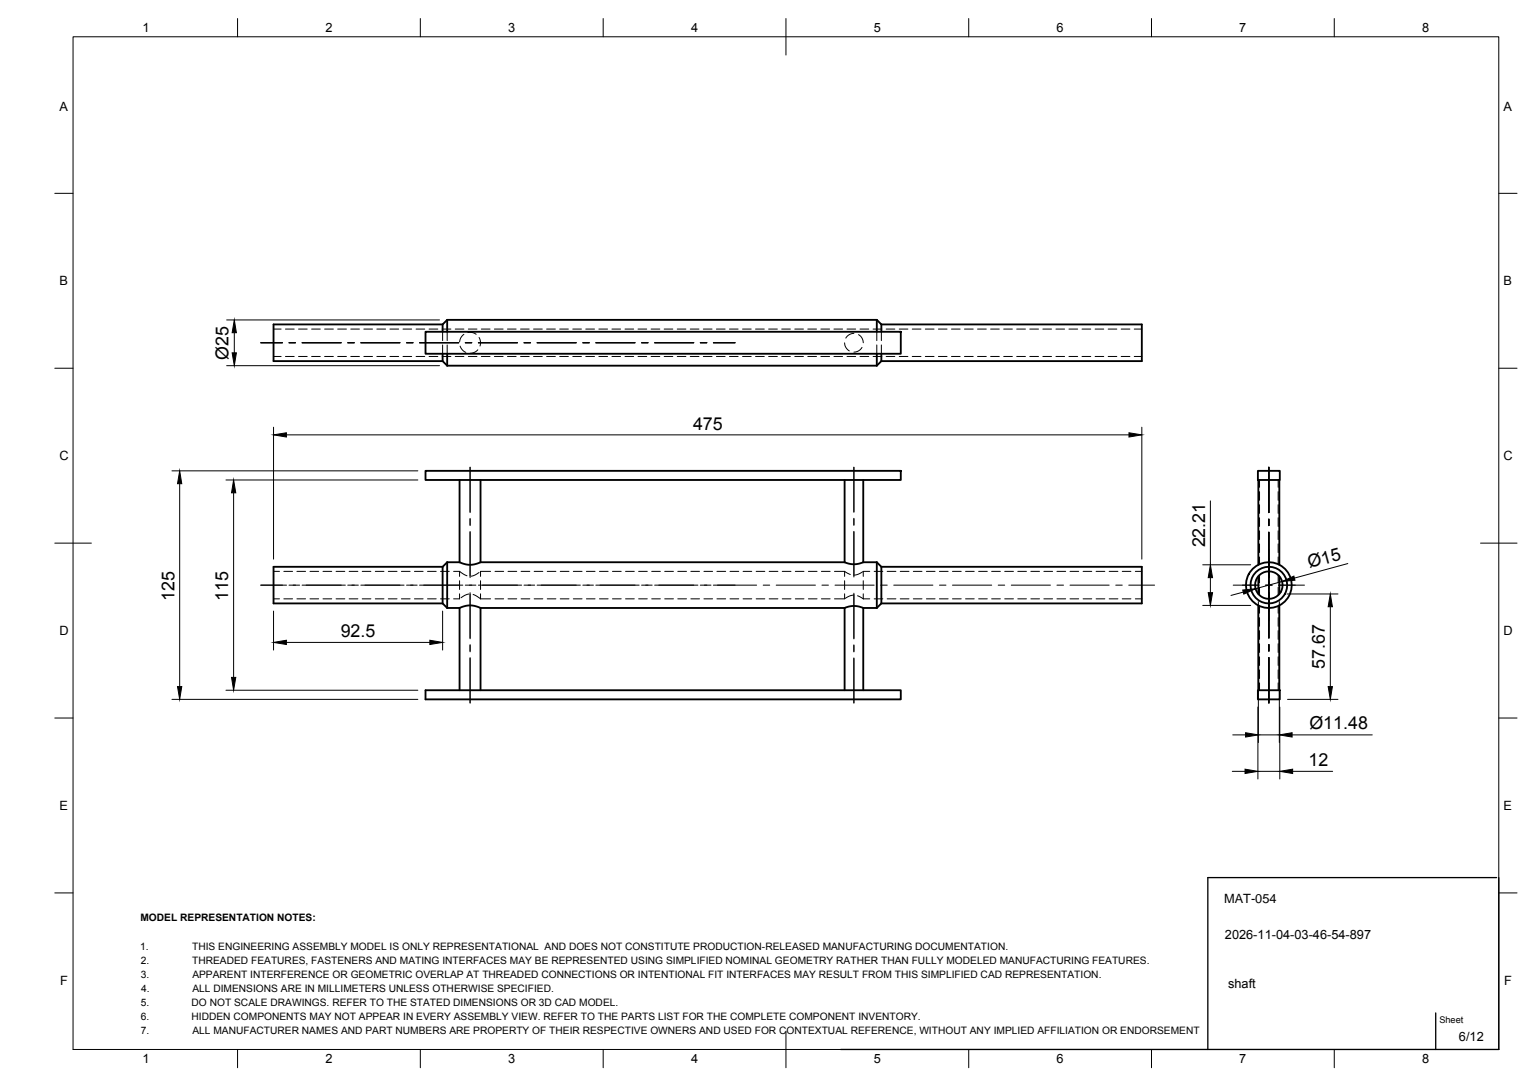
ISO-10303-21;
HEADER;
FILE_DESCRIPTION (('STEP AP214'),
    '1' );
FILE_NAME ('shaft.step',
    '2026-10-21T17:50:41',
    ( '' ),
    ( '' ),
    'SwSTEP 2.0',
    'SolidWorks 2026',
    '' );
FILE_SCHEMA (( 'AUTOMOTIVE_DESIGN' ));
ENDSEC;

DATA;
#16=VERTEX_POINT ( 'NONE', #3282 ) ;
#58=ADVANCED_FACE ( 'NONE', ( #14158 ), #33712, .T. ) ;
#109=VERTEX_POINT ( 'NONE', #18069 ) ;
#119=LINE ( 'NONE', #24139, #24170 ) ;
#137=CARTESIAN_POINT ( 'NONE',  ( -110.0810685637187021, 0.6776097359754142957, -12.48599830169775871 ) ) ;
#156=CARTESIAN_POINT ( 'NONE',  ( -109.6397584259853915, -2.159755022470678298, 7.184107906894084294 ) ) ;
#175=EDGE_CURVE ( 'NONE', #17916, #26514, #22520, .T. ) ;
#187=CIRCLE ( 'NONE', #747, 5.738084889453667792 ) ;
#195=ORIENTED_EDGE ( 'NONE', *, *, #25088, .F. ) ;
#198=CARTESIAN_POINT ( 'NONE',  ( 105.9801405217367147, 5.657025933901884684, 4.924586583110066584 ) ) ;
#251=ORIENTED_EDGE ( 'NONE', *, *, #8791, .F. ) ;
#257=CARTESIAN_POINT ( 'NONE',  ( 106.5104497542385928, -5.548707632555109015, -11.20129239819138967 ) ) ;
#273=EDGE_CURVE ( 'NONE', #17170, #26514, #10910, .T. ) ;
#275=CARTESIAN_POINT ( 'NONE',  ( -130.6469666100234406, 6.000000000000000000, 57.49999999999999289 ) ) ;
#291=CARTESIAN_POINT ( 'NONE',  ( -101.1657792522907329, 3.400963087932908024, 6.689628992625340942 ) ) ;
#341=CARTESIAN_POINT ( 'NONE',  ( -103.3057560645484045, -4.837552664684794834, 5.733718144795171945 ) ) ;
#348=VECTOR ( 'NONE', #16267, 1000.000000000000000 ) ;
#350=CARTESIAN_POINT ( 'NONE',  ( 105.0000000000000000, 0.000000000000000000, 60.00000000000000000 ) ) ;
#375=ORIENTED_EDGE ( 'NONE', *, *, #8635, .T. ) ;
#376=ADVANCED_FACE ( 'NONE', ( #22293 ), #33492, .T. ) ;
#380=ORIENTED_EDGE ( 'NONE', *, *, #13916, .T. ) ;
#435=EDGE_CURVE ( 'NONE', #18500, #31492, #4843, .T. ) ;
#441=DIRECTION ( 'NONE',  ( -1.000000000000000000, -0.000000000000000000, -0.000000000000000000 ) ) ;
#498=CARTESIAN_POINT ( 'NONE',  ( -100.0512976970618269, 1.336696757081942799, 12.43272095415539624 ) ) ;
#514=CARTESIAN_POINT ( 'NONE',  ( 110.5348319305551996, -1.563330414527343892, 7.345474502415979323 ) ) ;
#524=DIRECTION ( 'NONE',  ( -1.000000000000000000, 0.000000000000000000, 0.000000000000000000 ) ) ;
#549=VERTEX_POINT ( 'NONE', #28849 ) ;
#551=CARTESIAN_POINT ( 'NONE',  ( 103.6426013227723928, 5.578557642680240569, 5.013303406467239931 ) ) ;
#556=CARTESIAN_POINT ( 'NONE',  ( -104.3188479752188869, -5.080615126163384510, -11.42114788619746868 ) ) ;
#598=ORIENTED_EDGE ( 'NONE', *, *, #14200, .F. ) ;
#604=CARTESIAN_POINT ( 'NONE',  ( 100.0399502288726268, -2.891119662789794820, -12.16223328578254481 ) ) ;
#613=EDGE_LOOP ( 'NONE', ( #32797, #28941 ) ) ;
#636=ORIENTED_EDGE ( 'NONE', *, *, #31314, .F. ) ;
#648=CARTESIAN_POINT ( 'NONE',  ( 99.26191511054632599, 0.000000000000000000, 60.00000000000000000 ) ) ;
#696=FACE_OUTER_BOUND ( 'NONE', #25279, .T. ) ;
#715=CARTESIAN_POINT ( 'NONE',  ( -105.3381247832323027, -5.114954807106461665, 11.40557921924218832 ) ) ;
#729=CARTESIAN_POINT ( 'NONE',  ( 104.6074685613258168, 5.728031835420551943, 4.841551550731546527 ) ) ;
#730=SHAPE_DEFINITION_REPRESENTATION ( #21995, #18474 ) ;
#731=VERTEX_POINT ( 'NONE', #27233 ) ;
#733=CARTESIAN_POINT ( 'NONE',  ( -108.7324602969096645, -3.501388609494501036, -12.00022069954820836 ) ) ;
#747=AXIS2_PLACEMENT_3D ( 'NONE', #33040, #30386, #5986 ) ;
#781=CARTESIAN_POINT ( 'NONE',  ( 109.5465872284862741, -3.505526250977489156, -11.99932421786962067 ) ) ;
#811=CARTESIAN_POINT ( 'NONE',  ( 104.6049621835381487, -5.727834534852265236, -4.841784820303065118 ) ) ;
#826=CARTESIAN_POINT ( 'NONE',  ( 212.5000000000000000, 9.184850993605147944E-16, -7.500000000000000000 ) ) ;
#843=B_SPLINE_CURVE_WITH_KNOTS ( 'NONE', 3,
 ( #21300, #7758, #27153, #24466, #15972, #22001, #29835, #11154, #291, #21814, #5777, #7935, #18814, #32316, #10626, #26809, #19169, #2595, #18644, #2419, #21476, #13297, #10795, #24129, #13464, #16203, #32670, #8111, #18989, #24650, #8291, #5433, #16326, #27325, #32840, #2942 ),
 .UNSPECIFIED., .F., .F.,
 ( 4, 2, 2, 2, 2, 2, 2, 2, 2, 2, 2, 2, 2, 2, 2, 2, 2, 4 ),
 ( 4.603728119458012508E-18, 0.001035696236907480625, 0.002071392473814956912, 0.003107088710722432333, 0.004142784947629908621, 0.005178481184537384041, 0.006214177421444859462, 0.007249873658352335749, 0.007767721776806054378, 0.008285569895259772139, 0.009321266132167249294, 0.01035696236907472818, 0.01087481048752844855, 0.01139265860598217064, 0.01242835484288958188, 0.01449974731670443211, 0.01553544355361186069, 0.01657113979051928407 ),
 .UNSPECIFIED. ) ;
#846=CARTESIAN_POINT ( 'NONE',  ( -100.4098818337750885, 2.281765576240580629, 12.29396198687797259 ) ) ;
#896=CARTESIAN_POINT ( 'NONE',  ( -110.0477662801539935, -0.8438318447813555334, 12.47259309357265522 ) ) ;
#900=ORIENTED_EDGE ( 'NONE', *, *, #18867, .T. ) ;
#907=CARTESIAN_POINT ( 'NONE',  ( 212.5000000000000000, 0.000000000000000000, 0.000000000000000000 ) ) ;
#912=CARTESIAN_POINT ( 'NONE',  ( -100.9389840009208825, -3.127506413740531510, -12.10571963949988650 ) ) ;
#946=ORIENTED_EDGE ( 'NONE', *, *, #3678, .T. ) ;
#972=CARTESIAN_POINT ( 'NONE',  ( -105.0000000000000000, 0.000000000000000000, 60.00000000000000000 ) ) ;
#1030=DIRECTION ( 'NONE',  ( -0.000000000000000000, -0.000000000000000000, -1.000000000000000000 ) ) ;
#1097=CARTESIAN_POINT ( 'NONE',  ( 105.0000000000000000, 0.000000000000000000, -57.49999999999999289 ) ) ;
#1124=ORIENTED_EDGE ( 'NONE', *, *, #19366, .T. ) ;
#1125=VERTEX_POINT ( 'NONE', #275 ) ;
#1149=CARTESIAN_POINT ( 'NONE',  ( -130.6469666100234406, 6.000000000000000000, 62.49999999999999289 ) ) ;
#1151=CARTESIAN_POINT ( 'NONE',  ( 104.2139989449238442, 5.687433884741868617, -4.889179432777876144 ) ) ;
#1164=CARTESIAN_POINT ( 'NONE',  ( 99.46516806944471512, -1.563330414527343892, -7.345474502415979323 ) ) ;
#1221=CARTESIAN_POINT ( 'NONE',  ( 212.5000000000000000, 0.000000000000000000, 10.00000000000000000 ) ) ;
#1229=CARTESIAN_POINT ( 'NONE',  ( 109.1843660233815996, 3.930740943550895761, 11.86668706373619386 ) ) ;
#1239=CARTESIAN_POINT ( 'NONE',  ( -130.6469666100234406, -6.000000000000000000, 57.49999999999999289 ) ) ;
#1255=ADVANCED_FACE ( 'NONE', ( #27847 ), #16878, .T. ) ;
#1261=CARTESIAN_POINT ( 'NONE',  ( -101.8768327269408189, -4.064293880962482675, -11.82242856119474439 ) ) ;
#1278=VECTOR ( 'NONE', #1030, 1000.000000000000000 ) ;
#1309=DIRECTION ( 'NONE',  ( -0.000000000000000000, -0.000000000000000000, -1.000000000000000000 ) ) ;
#1344=CARTESIAN_POINT ( 'NONE',  ( 99.58236139071918558, -1.928835813323004800, -7.257044673176061167 ) ) ;
#1374=CARTESIAN_POINT ( 'NONE',  ( -109.4269239543884851, 2.567831768330360642, 12.23432884111322316 ) ) ;
#1387=FACE_OUTER_BOUND ( 'NONE', #26140, .T. ) ;
#1411=CARTESIAN_POINT ( 'NONE',  ( 212.5000000000000000, 0.000000000000000000, 0.000000000000000000 ) ) ;
#1415=CARTESIAN_POINT ( 'NONE',  ( 99.26191511054632599, 0.000000000000000000, 57.49999999999999289 ) ) ;
#1461=AXIS2_PLACEMENT_3D ( 'NONE', #27978, #24945, #19458 ) ;
#1513=CARTESIAN_POINT ( 'NONE',  ( 99.26191511054628336, -0.3983872338823410408, -7.499999999999998224 ) ) ;
#1524=EDGE_CURVE ( 'NONE', #14561, #13528, #33154, .T. ) ;
#1556=CARTESIAN_POINT ( 'NONE',  ( 105.7529209506896422, -5.691643476845047012, 11.12904465084466565 ) ) ;
#1557=EDGE_LOOP ( 'NONE', ( #29453, #13377 ) ) ;
#1560=DIRECTION ( 'NONE',  ( -1.000000000000000000, 0.000000000000000000, 0.000000000000000000 ) ) ;
#1572=CIRCLE ( 'NONE', #10080, 10.00000000000000000 ) ;
#1596=ORIENTED_EDGE ( 'NONE', *, *, #34606, .T. ) ;
#1648=ORIENTED_EDGE ( 'NONE', *, *, #30047, .F. ) ;
#1663=DIRECTION ( 'NONE',  ( 0.000000000000000000, 0.000000000000000000, 1.000000000000000000 ) ) ;
#1723=CARTESIAN_POINT ( 'NONE',  ( 104.2381396081001412, -5.690476701307018104, 11.12964202013672299 ) ) ;
#1748=LINE ( 'NONE', #9245, #34250 ) ;
#1761=EDGE_CURVE ( 'NONE', #2593, #32910, #21774, .T. ) ;
#1769=CARTESIAN_POINT ( 'NONE',  ( 105.1990410865049057, -5.738006884272855324, 4.829624934769205069 ) ) ;
#1774=FACE_OUTER_BOUND ( 'NONE', #27919, .T. ) ;
#1789=AXIS2_PLACEMENT_3D ( 'NONE', #23876, #11559, #21871 ) ;
#1808=CARTESIAN_POINT ( 'NONE',  ( 110.5382509904757313, 1.550744593849150865, 7.348056298371736794 ) ) ;
#1823=CARTESIAN_POINT ( 'NONE',  ( 119.9999999999998295, 1.224646799147353256E-15, -10.00000000000000000 ) ) ;
#1835=CARTESIAN_POINT ( 'NONE',  ( 110.3448550603046527, 2.096151729099205774, -7.203423290846323823 ) ) ;
#1837=CARTESIAN_POINT ( 'NONE',  ( -108.8342207477093240, 3.400963087932895146, -6.689628992625347159 ) ) ;
#1843=( LENGTH_UNIT ( ) NAMED_UNIT ( * ) SI_UNIT ( .MILLI., .METRE. ) );
#1867=ORIENTED_EDGE ( 'NONE', *, *, #17479, .T. ) ;
#1872=CARTESIAN_POINT ( 'NONE',  ( 99.26191511054632599, 1.643815732525060864E-21, 12.50000000000000000 ) ) ;
#1894=CARTESIAN_POINT ( 'NONE',  ( 102.4434507907919141, -5.150622582557323526, 11.39062369188951607 ) ) ;
#1941=LINE ( 'NONE', #18343, #30370 ) ;
#1942=CARTESIAN_POINT ( 'NONE',  ( 103.0920869195258689, -5.424061631995436450, 5.183681401394261812 ) ) ;
#1990=EDGE_CURVE ( 'NONE', #17916, #31492, #14309, .T. ) ;
#2015=CARTESIAN_POINT ( 'NONE',  ( 109.5206256355305214, 3.553124229080486085, -6.613494096335986505 ) ) ;
#2017=CARTESIAN_POINT ( 'NONE',  ( -108.1229279508730627, 4.063889691276223459, -6.307349793299454888 ) ) ;
#2021=CARTESIAN_POINT ( 'NONE',  ( 110.7380848894536598, 7.027143731242819742E-16, -12.50000000000000000 ) ) ;
#2033=ORIENTED_EDGE ( 'NONE', *, *, #1761, .T. ) ;
#2037=EDGE_CURVE ( 'NONE', #109, #31150, #1941, .T. ) ;
#2123=CARTESIAN_POINT ( 'NONE',  ( 104.6067242497968834, -5.728011724833245388, 4.841576811596270069 ) ) ;
#2152=DIRECTION ( 'NONE',  ( 1.000000000000000000, 0.000000000000000000, 0.000000000000000000 ) ) ;
#2156=ADVANCED_FACE ( 'NONE', ( #32197 ), #18526, .T. ) ;
#2162=CONICAL_SURFACE ( 'NONE', #12977, 12.50000000000000000, 0.7853981633974431720 ) ;
#2166=ORIENTED_EDGE ( 'NONE', *, *, #23931, .T. ) ;
#2183=CARTESIAN_POINT ( 'NONE',  ( -130.6469666100234406, 6.000000000000000000, 62.49999999999999289 ) ) ;
#2184=CARTESIAN_POINT ( 'NONE',  ( 212.5000000000000000, 0.000000000000000000, 7.500000000000000000 ) ) ;
#2200=DIRECTION ( 'NONE',  ( 0.000000000000000000, 0.000000000000000000, 1.000000000000000000 ) ) ;
#2243=DIRECTION ( 'NONE',  ( 0.000000000000000000, -0.000000000000000000, 1.000000000000000000 ) ) ;
#2252=CARTESIAN_POINT ( 'NONE',  ( -101.1679389503612612, -3.403480489512942686, -6.688370467007151099 ) ) ;
#2256=ORIENTED_EDGE ( 'NONE', *, *, #9336, .T. ) ;
#2269=CYLINDRICAL_SURFACE ( 'NONE', #31981, 5.738084889453667792 ) ;
#2270=ORIENTED_EDGE ( 'NONE', *, *, #27716, .T. ) ;
#2272=EDGE_CURVE ( 'NONE', #23099, #33855, #19613, .T. ) ;
#2287=CARTESIAN_POINT ( 'NONE',  ( -105.0000000000000000, 0.000000000000000000, 60.00000000000000000 ) ) ;
#2288=CARTESIAN_POINT ( 'NONE',  ( 99.27229867161369725, -0.3974226492620277496, 7.492047161373153408 ) ) ;
#2290=AXIS2_PLACEMENT_3D ( 'NONE', #22014, #33027, #29848 ) ;
#2313=DIRECTION ( 'NONE',  ( 0.000000000000000000, 0.000000000000000000, -1.000000000000000000 ) ) ;
#2323=CARTESIAN_POINT ( 'NONE',  ( 129.3530333899765594, -6.000000000000000000, -57.49999999999999289 ) ) ;
#2328=CARTESIAN_POINT ( 'NONE',  ( 110.6969072286498204, 0.7888478034546075879, 7.468363897292212172 ) ) ;
#2352=LINE ( 'NONE', #2184, #18636 ) ;
#2362=CARTESIAN_POINT ( 'NONE',  ( 105.1857752594875990, 5.738231822805251348, -11.10507521702373879 ) ) ;
#2419=CARTESIAN_POINT ( 'NONE',  ( -105.3457392332551734, 5.115129524682074269, 5.485020507536670031 ) ) ;
#2422=CARTESIAN_POINT ( 'NONE',  ( -105.8662310357297400, -5.044029065977393422, -5.550668370081900171 ) ) ;
#2430=EDGE_CURVE ( 'NONE', #34071, #27140, #17962, .T. ) ;
#2441=CARTESIAN_POINT ( 'NONE',  ( 99.45027429990390999, 1.507575458593797046, 12.41447922803859072 ) ) ;
#2447=CARTESIAN_POINT ( 'NONE',  ( -109.8484943653665056, 1.663653002832651051, -12.39274845084345600 ) ) ;
#2466=CARTESIAN_POINT ( 'NONE',  ( 107.5858466720334974, -5.135784989587515170, 5.469495349232144754 ) ) ;
#2471=EDGE_CURVE ( 'NONE', #26514, #17916, #10433, .T. ) ;
#2521=DIRECTION ( 'NONE',  ( 0.000000000000000000, -0.000000000000000000, 1.000000000000000000 ) ) ;
#2529=B_SPLINE_CURVE_WITH_KNOTS ( 'NONE', 3,
 ( #34558, #15895, #2328, #1808, #24036, #23523, #34923, #20855, #10539, #26366, #21391, #23702, #21029, #31866, #32237, #25093, #13724, #198, #16768, #13905, #18903, #729, #2688, #24748, #551, #19429, #16418, #8381, #14263, #11063, #11595, #5689, #16949, #11237, #2854, #8021, #16589, #32932, #32577, #22445, #8200, #11406, #22265, #5348, #24561 ),
 .UNSPECIFIED., .F., .F.,
 ( 4, 2, 2, 2, 2, 2, 2, 2, 2, 2, 1, 2, 2, 2, 2, 2, 2, 2, 2, 2, 2, 2, 4 ),
 ( 3.984693255910324139E-19, 0.001177949164446570477, 0.002355898328893140520, 0.003533847493339711213, 0.004711796657786281907, 0.005889745822232853034, 0.007067694986679424161, 0.007656669568902727506, 0.008245644151126031718, 0.008834618733349335062, 0.009423593315572640142, 0.01001256789779594349, 0.01060154248001924683, 0.01119051706224255191, 0.01177949164446585525, 0.01295744080891246194, 0.01413538997335907210, 0.01531333913780567879, 0.01590231372002897173, 0.01649128830225226466, 0.01708026288447555760, 0.01766923746669885054, 0.01884718663114543988 ),
 .UNSPECIFIED. ) ;
#2545=EDGE_LOOP ( 'NONE', ( #1596, #26188, #15712, #31943 ) ) ;
#2585=EDGE_CURVE ( 'NONE', #27140, #731, #11334, .T. ) ;
#2593=VERTEX_POINT ( 'NONE', #13822 ) ;
#2595=CARTESIAN_POINT ( 'NONE',  ( -104.6485238499209203, 5.105882603317797752, 5.493682664683364081 ) ) ;
#2600=CARTESIAN_POINT ( 'NONE',  ( -107.3019298601570881, -4.579683091146231178, -5.941712070794213929 ) ) ;
#2648=CARTESIAN_POINT ( 'NONE',  ( -100.0251193558530076, -1.201525761660788838, 7.405089084531746302 ) ) ;
#2688=CARTESIAN_POINT ( 'NONE',  ( 104.2155338827948867, 5.687621871124707518, 4.888959764314519063 ) ) ;
#2712=CARTESIAN_POINT ( 'NONE',  ( -102.4161755605319968, 4.417479313406522223, -6.061799023038633827 ) ) ;
#2735=ORIENTED_EDGE ( 'NONE', *, *, #2430, .T. ) ;
#2770=CARTESIAN_POINT ( 'NONE',  ( 129.3530333899765594, 6.000000000000000000, 62.49999999999999289 ) ) ;
#2785=AXIS2_PLACEMENT_3D ( 'NONE', #972, #32986, #28194 ) ;
#2789=ORIENTED_EDGE ( 'NONE', *, *, #23686, .F. ) ;
#2797=CARTESIAN_POINT ( 'NONE',  ( -107.5694449394638070, 4.435438170924840939, -11.68828588916098532 ) ) ;
#2811=VERTEX_POINT ( 'NONE', #7719 ) ;
#2816=CARTESIAN_POINT ( 'NONE',  ( -104.3033539127188902, -5.070312235224276876, 5.526528498279830615 ) ) ;
#2854=CARTESIAN_POINT ( 'NONE',  ( 100.1670491183068208, 3.098707215121725422, 6.832002823648420708 ) ) ;
#2896=B_SPLINE_CURVE_WITH_KNOTS ( 'NONE', 3,
 ( #10136, #15318, #2288, #31663, #34341, #7271, #21353, #16020, #4425, #4775, #15851, #34694, #15490, #23662, #29536, #1942, #26854, #20993, #18694, #2123, #7447, #1769, #15671, #21168, #7629, #18527, #29361, #2466, #9783, #20647, #4956, #31490, #12646, #23481, #9960, #20819, #30408, #27035, #514, #22049, #32365, #32893 ),
 .UNSPECIFIED., .F., .F.,
 ( 4, 2, 2, 2, 2, 2, 2, 2, 2, 2, 2, 2, 2, 2, 2, 2, 2, 2, 2, 2, 4 ),
 ( 0.01884718663114543988, 0.01943499450852638824, 0.02002280238590734007, 0.02119841814066924027, 0.02237403389543114046, 0.02354964965019304066, 0.02472526540495494085, 0.02590088115971684452, 0.02707649691447874471, 0.02766430479185969654, 0.02825211266924064490, 0.02883992054662159674, 0.02942772842400254510, 0.03060334417876444529, 0.03177895993352634896, 0.03295457568828825262, 0.03413019144305015629, 0.03471799932043109771, 0.03530580719781203913, 0.03648142295257392198, 0.03765703870733580483 ),
 .UNSPECIFIED. ) ;
#2942=CARTESIAN_POINT ( 'NONE',  ( -110.1150203881707910, -1.604996202923496961E-20, 7.500000000000000000 ) ) ;
#3038=ADVANCED_FACE ( 'NONE', ( #21963 ), #16109, .T. ) ;
#3061=CARTESIAN_POINT ( 'NONE',  ( -100.5621347894176836, 2.632420417224713649, -7.052679658646594518 ) ) ;
#3091=CARTESIAN_POINT ( 'NONE',  ( 109.1840482152002210, -3.931125184197653333, -11.86656790805995243 ) ) ;
#3092=CARTESIAN_POINT ( 'NONE',  ( -262.5000000000000000, 0.000000000000000000, 10.00000000000000000 ) ) ;
#3100=DIRECTION ( 'NONE',  ( -0.000000000000000000, -0.000000000000000000, -1.000000000000000000 ) ) ;
#3148=VECTOR ( 'NONE', #24505, 1000.000000000000000 ) ;
#3171=CARTESIAN_POINT ( 'NONE',  ( -104.8237380854588707, -5.114955647091109725, 5.485182652933519698 ) ) ;
#3224=CARTESIAN_POINT ( 'NONE',  ( 129.3530333899765594, 6.000000000000000000, 57.49999999999999289 ) ) ;
#3229=DIRECTION ( 'NONE',  ( -1.000000000000000000, 0.000000000000000000, 0.000000000000000000 ) ) ;
#3253=ADVANCED_FACE ( 'NONE', ( #31540 ), #2162, .T. ) ;
#3260=VECTOR ( 'NONE', #24940, 1000.000000000000000 ) ;
#3277=FACE_OUTER_BOUND ( 'NONE', #12265, .T. ) ;
#3282=CARTESIAN_POINT ( 'NONE',  ( 212.5000000000000000, 9.184850993605147944E-16, -7.500000000000000000 ) ) ;
#3375=CARTESIAN_POINT ( 'NONE',  ( -99.88497961182923746, -0.3417625387765687028, 12.50000000000000178 ) ) ;
#3389=CARTESIAN_POINT ( 'NONE',  ( -100.4172690689928373, -2.278159677709879816, -12.29156386665007439 ) ) ;
#3427=ORIENTED_EDGE ( 'NONE', *, *, #26103, .F. ) ;
#3443=CARTESIAN_POINT ( 'NONE',  ( 110.7380848894536598, 7.027127293105233764E-16, 60.00000000000000000 ) ) ;
#3447=CARTESIAN_POINT ( 'NONE',  ( 100.4805201888165982, 3.554679846740550264, -6.612701241491620863 ) ) ;
#3454=EDGE_LOOP ( 'NONE', ( #14838, #22488, #7870, #3427 ) ) ;
#3456=DIRECTION ( 'NONE',  ( 1.000000000000000000, 0.000000000000000000, 0.000000000000000000 ) ) ;
#3482=VECTOR ( 'NONE', #7845, 1000.000000000000000 ) ;
#3501=CARTESIAN_POINT ( 'NONE',  ( -99.88497961182922324, 0.3420146137956281973, 12.50000000000000178 ) ) ;
#3566=CARTESIAN_POINT ( 'NONE',  ( -110.1150203881707910, 0.000000000000000000, 60.00000000000000000 ) ) ;
#3568=ORIENTED_EDGE ( 'NONE', *, *, #13544, .F. ) ;
#3602=ORIENTED_EDGE ( 'NONE', *, *, #11901, .T. ) ;
#3640=CARTESIAN_POINT ( 'NONE',  ( 105.1945178213486116, -5.738162003225207641, -4.829440634198706839 ) ) ;
#3665=ORIENTED_EDGE ( 'NONE', *, *, #25088, .T. ) ;
#3676=CARTESIAN_POINT ( 'NONE',  ( -100.9388899323377586, 3.127595108844668292, 12.10573782681415267 ) ) ;
#3678=EDGE_CURVE ( 'NONE', #21237, #12316, #12133, .T. ) ;
#3698=EDGE_CURVE ( 'NONE', #20721, #16671, #31190, .T. ) ;
#3704=EDGE_CURVE ( 'NONE', #549, #17916, #30462, .T. ) ;
#3729=CARTESIAN_POINT ( 'NONE',  ( -101.2675397030902928, -3.501388609494501036, 12.00022069954821013 ) ) ;
#3793=FACE_OUTER_BOUND ( 'NONE', #613, .T. ) ;
#3818=CARTESIAN_POINT ( 'NONE',  ( 104.0188950037896660, -5.656875047978680904, -4.924762495648698390 ) ) ;
#3848=CARTESIAN_POINT ( 'NONE',  ( -102.4305550605362214, 4.435438170924840939, 11.68828588916098887 ) ) ;
#3850=CIRCLE ( 'NONE', #32837, 12.50000000000000000 ) ;
#3852=ADVANCED_FACE ( 'NONE', ( #1774 ), #18178, .F. ) ;
#3855=DIRECTION ( 'NONE',  ( 0.000000000000000000, 0.000000000000000000, -1.000000000000000000 ) ) ;
#3870=VERTEX_POINT ( 'NONE', #16207 ) ;
#3881=CARTESIAN_POINT ( 'NONE',  ( 105.7609509841301190, 5.700015625666662089, 11.12505441474362655 ) ) ;
#3894=CARTESIAN_POINT ( 'NONE',  ( -109.6555751755425376, -2.125365432952319278, 12.31898464336051902 ) ) ;
#3908=CARTESIAN_POINT ( 'NONE',  ( -108.8452008526440551, -3.377194313163045969, -12.03587146382073669 ) ) ;
#3925=VERTEX_POINT ( 'NONE', #13524 ) ;
#3931=AXIS2_PLACEMENT_3D ( 'NONE', #31931, #24093, #7546 ) ;
#3968=LINE ( 'NONE', #12364, #30439 ) ;
#3983=VERTEX_POINT ( 'NONE', #26861 ) ;
#3985=CARTESIAN_POINT ( 'NONE',  ( 105.9791845165408546, -5.657186516187210579, -4.924400946180165661 ) ) ;
#3986=ORIENTED_EDGE ( 'NONE', *, *, #14193, .T. ) ;
#4021=CARTESIAN_POINT ( 'NONE',  ( 105.0000000000000000, 0.000000000000000000, 57.49999999999999289 ) ) ;
#4030=EDGE_CURVE ( 'NONE', #26496, #1125, #12563, .T. ) ;
#4034=EDGE_LOOP ( 'NONE', ( #29464, #29518, #34962, #1124, #31204, #11890, #26411, #30818, #32095, #20216, #1648, #14061 ) ) ;
#4050=CARTESIAN_POINT ( 'NONE',  ( 109.9700946220824278, 2.891935069322400853, 12.16509469334829774 ) ) ;
#4063=CARTESIAN_POINT ( 'NONE',  ( -104.6638623058952078, -5.115085776248456284, 11.40552048381710115 ) ) ;
#4076=ORIENTED_EDGE ( 'NONE', *, *, #19368, .T. ) ;
#4091=FACE_OUTER_BOUND ( 'NONE', #26156, .T. ) ;
#4110=EDGE_CURVE ( 'NONE', #19142, #3983, #9704, .T. ) ;
#4117=PLANE ( 'NONE',  #17652 ) ;
#4132=CARTESIAN_POINT ( 'NONE',  ( -110.1150203881707910, 0.000000000000000000, 60.00000000000000000 ) ) ;
#4148=CARTESIAN_POINT ( 'NONE',  ( -109.5740446912284938, 2.313922778582933493, -7.141321738367096827 ) ) ;
#4209=CARTESIAN_POINT ( 'NONE',  ( 100.0393311773591023, -2.890043774996763570, 12.16248655421354385 ) ) ;
#4230=CARTESIAN_POINT ( 'NONE',  ( 105.3850032505120424, 5.737785766176326518, 11.10530569653546706 ) ) ;
#4237=ORIENTED_EDGE ( 'NONE', *, *, #2585, .F. ) ;
#4238=CARTESIAN_POINT ( 'NONE',  ( -110.1150203881707910, -7.176976838982289656E-16, -12.50000000000000000 ) ) ;
#4239=ADVANCED_FACE ( 'NONE', ( #26599 ), #13266, .F. ) ;
#4253=CARTESIAN_POINT ( 'NONE',  ( -109.0426547331720855, -3.150844840328208996, 6.812360382669037762 ) ) ;
#4271=VECTOR ( 'NONE', #19526, 1000.000000000000000 ) ;
#4299=EDGE_CURVE ( 'NONE', #7716, #14308, #7768, .T. ) ;
#4301=DIRECTION ( 'NONE',  ( 1.000000000000000000, -0.000000000000000000, -0.000000000000000000 ) ) ;
#4311=ORIENTED_EDGE ( 'NONE', *, *, #4030, .F. ) ;
#4322=CARTESIAN_POINT ( 'NONE',  ( -103.3138142205062024, 4.840548292904077066, -5.731216124222060060 ) ) ;
#4342=AXIS2_PLACEMENT_3D ( 'NONE', #20835, #9464, #18016 ) ;
#4372=AXIS2_PLACEMENT_3D ( 'NONE', #28974, #10107, #7417 ) ;
#4377=ORIENTED_EDGE ( 'NONE', *, *, #34606, .F. ) ;
#4381=CARTESIAN_POINT ( 'NONE',  ( 100.6898240025452793, -3.792433597769625298, 11.91175651985687267 ) ) ;
#4384=DIRECTION ( 'NONE',  ( -1.000000000000000000, 0.000000000000000000, 0.000000000000000000 ) ) ;
#4394=DIRECTION ( 'NONE',  ( -1.000000000000000000, -0.000000000000000000, -0.000000000000000000 ) ) ;
#4425=CARTESIAN_POINT ( 'NONE',  ( 100.0637405348225144, -2.948796715283049874, 6.904248079351286371 ) ) ;
#4443=VECTOR ( 'NONE', #1560, 1000.000000000000000 ) ;
#4480=DIRECTION ( 'NONE',  ( -1.000000000000000000, -0.000000000000000000, -0.000000000000000000 ) ) ;
#4491=CARTESIAN_POINT ( 'NONE',  ( 105.3925314386741405, 5.728031835420551943, -4.841551550731546527 ) ) ;
#4496=CARTESIAN_POINT ( 'NONE',  ( 104.6149967494879149, 5.737785766176327407, -11.10530569653546706 ) ) ;
#4539=DIRECTION ( 'NONE',  ( 1.000000000000000000, 0.000000000000000000, 0.000000000000000000 ) ) ;
#4546=CARTESIAN_POINT ( 'NONE',  ( 99.45057497126383339, -1.507735446164281790, 12.41434713890700969 ) ) ;
#4553=PLANE ( 'NONE',  #27888 ) ;
#4568=CARTESIAN_POINT ( 'NONE',  ( 99.85824206759374988, 2.553994279224884423, 12.23746534924524632 ) ) ;
#4587=VECTOR ( 'NONE', #9875, 1000.000000000000000 ) ;
#4622=ADVANCED_FACE ( 'NONE', ( #15540 ), #15909, .T. ) ;
#4661=CARTESIAN_POINT ( 'NONE',  ( -109.9413161124788445, 1.365406536427363315, -7.382450522560829675 ) ) ;
#4665=CARTESIAN_POINT ( 'NONE',  ( 109.5543437205592170, 3.510468032099188118, -12.00123740321143728 ) ) ;
#4676=STYLED_ITEM('',(#35275),#34055);
#4693=ORIENTED_EDGE ( 'NONE', *, *, #4299, .T. ) ;
#4721=ADVANCED_FACE ( 'NONE', ( #16429 ), #13741, .T. ) ;
#4731=CARTESIAN_POINT ( 'NONE',  ( -100.3602415740146228, -2.159755022470677854, -7.184107906894083406 ) ) ;
#4746=EDGE_LOOP ( 'NONE', ( #5289, #375, #12548, #2256 ) ) ;
#4748=CARTESIAN_POINT ( 'NONE',  ( 99.26191511054629757, 0.3793982372081725063, 12.50000000000000000 ) ) ;
#4754=ORIENTED_EDGE ( 'NONE', *, *, #20666, .T. ) ;
#4775=CARTESIAN_POINT ( 'NONE',  ( 100.4825637827005238, -3.557362730766958858, 6.611294427798556583 ) ) ;
#4806=CARTESIAN_POINT ( 'NONE',  ( 212.5000000000000000, 0.000000000000000000, 0.000000000000000000 ) ) ;
#4815=ORIENTED_EDGE ( 'NONE', *, *, #7136, .T. ) ;
#4840=AXIS2_PLACEMENT_3D ( 'NONE', #25035, #9210, #3855 ) ;
#4843=CIRCLE ( 'NONE', #1461, 7.500000000000000000 ) ;
#4844=CYLINDRICAL_SURFACE ( 'NONE', #6075, 5.115020388170798959 ) ;
#4851=CARTESIAN_POINT ( 'NONE',  ( 100.0299053779175580, 2.891935069322401297, -12.16509469334830307 ) ) ;
#4905=CARTESIAN_POINT ( 'NONE',  ( 110.4382027763065963, -1.869077253746796341, 12.36451290817386450 ) ) ;
#4910=CARTESIAN_POINT ( 'NONE',  ( -109.8286890707746011, -1.696008709688487048, -7.307621933264762504 ) ) ;
#4934=CIRCLE ( 'NONE', #14708, 12.50000000000000000 ) ;
#4956=CARTESIAN_POINT ( 'NONE',  ( 108.7726925648793070, -4.338569679229816067, 6.125236864567445316 ) ) ;
#4987=VECTOR ( 'NONE', #27292, 1000.000000000000000 ) ;
#5007=ORIENTED_EDGE ( 'NONE', *, *, #1761, .F. ) ;
#5075=CARTESIAN_POINT ( 'NONE',  ( 129.3530333899765594, 6.000000000000000000, 62.49999999999999289 ) ) ;
#5089=CARTESIAN_POINT ( 'NONE',  ( -99.95520222082589612, -0.8621751556914646342, -7.452240479933208483 ) ) ;
#5110=CARTESIAN_POINT ( 'NONE',  ( -103.6627159225451180, 4.948560684155824951, -11.47897987543853660 ) ) ;
#5112=CIRCLE ( 'NONE', #14244, 12.50000000000000000 ) ;
#5143=LINE ( 'NONE', #31844, #34170 ) ;
#5155=CARTESIAN_POINT ( 'NONE',  ( -262.5000000000000000, 0.000000000000000000, 0.000000000000000000 ) ) ;
#5170=AXIS2_PLACEMENT_3D ( 'NONE', #4806, #7657, #2313 ) ;
#5188=CARTESIAN_POINT ( 'NONE',  ( -105.0000000000000000, 0.000000000000000000, 60.00000000000000000 ) ) ;
#5190=LINE ( 'NONE', #32260, #9834 ) ;
#5223=DIRECTION ( 'NONE',  ( -1.000000000000000000, 0.000000000000000000, 0.000000000000000000 ) ) ;
#5225=LINE ( 'NONE', #10773, #6000 ) ;
#5252=ORIENTED_EDGE ( 'NONE', *, *, #27717, .F. ) ;
#5258=CARTESIAN_POINT ( 'NONE',  ( -102.7050928880580329, -4.583230167788444831, -5.938965658480648280 ) ) ;
#5273=DIRECTION ( 'NONE',  ( 1.000000000000000000, -0.000000000000000000, -0.000000000000000000 ) ) ;
#5289=ORIENTED_EDGE ( 'NONE', *, *, #25264, .T. ) ;
#5303=DIRECTION ( 'NONE',  ( -0.000000000000000000, -0.000000000000000000, -1.000000000000000000 ) ) ;
#5304=CARTESIAN_POINT ( 'NONE',  ( -109.5657259334022342, -2.311989032590052950, 7.136426621730641351 ) ) ;
#5329=ORIENTED_EDGE ( 'NONE', *, *, #27121, .F. ) ;
#5348=CARTESIAN_POINT ( 'NONE',  ( 99.26191511054628336, 0.3953117532656757471, 7.500000000000019540 ) ) ;
#5406=CARTESIAN_POINT ( 'NONE',  ( 100.1361914745664592, -3.050121699374163331, -12.12320065612944120 ) ) ;
#5433=CARTESIAN_POINT ( 'NONE',  ( -109.8376268937510218, 1.695881020439944598, 7.312931660397135047 ) ) ;
#5466=CARTESIAN_POINT ( 'NONE',  ( -100.1508892704537459, 1.661471846880724357, -12.39299840842996048 ) ) ;
#5482=CARTESIAN_POINT ( 'NONE',  ( -110.0713174531508827, -0.6892679340434131330, 7.470251853870532699 ) ) ;
#5515=VERTEX_POINT ( 'NONE', #24833 ) ;
#5530=CARTESIAN_POINT ( 'NONE',  ( 110.7380848894536598, -4.118294838564020743E-16, 7.500000000000000000 ) ) ;
#5544=CARTESIAN_POINT ( 'NONE',  ( -100.0603537787683592, 1.371756618311863685, -7.381329779211299957 ) ) ;
#5573=CARTESIAN_POINT ( 'NONE',  ( 99.56179722369340368, -1.869077253746796785, -12.36451290817385917 ) ) ;
#5631=CARTESIAN_POINT ( 'NONE',  ( -100.4147610035674916, 2.273103392716669724, -12.29250028061669120 ) ) ;
#5650=CARTESIAN_POINT ( 'NONE',  ( -99.88497961182920903, -0.3503014826537200754, 7.499999999999999112 ) ) ;
#5689=CARTESIAN_POINT ( 'NONE',  ( 101.2209703486791881, 4.332787265952012135, 6.129206022554251732 ) ) ;
#5717=CARTESIAN_POINT ( 'NONE',  ( -102.2775073974855644, 4.333302303957503376, -6.122453330911794112 ) ) ;
#5742=CARTESIAN_POINT ( 'NONE',  ( 109.9606688226409119, -2.890043774996748027, -12.16248655421355451 ) ) ;
#5777=CARTESIAN_POINT ( 'NONE',  ( -101.8770720491269088, 4.063889691276224347, 6.307349793299453111 ) ) ;
#5805=CARTESIAN_POINT ( 'NONE',  ( 127.4999999999999147, 0.000000000000000000, 12.50000000000000000 ) ) ;
#5809=CARTESIAN_POINT ( 'NONE',  ( -106.3372840774548536, 4.948560684155827616, 11.47897987543853837 ) ) ;
#5827=CARTESIAN_POINT ( 'NONE',  ( -106.6861982456198916, -4.840385614786934632, 5.731315639859859701 ) ) ;
#5834=FACE_OUTER_BOUND ( 'NONE', #3454, .T. ) ;
#5885=LINE ( 'NONE', #3224, #9152 ) ;
#5927=CARTESIAN_POINT ( 'NONE',  ( 101.4955157918503375, -4.558675695222540902, -11.64123453730966951 ) ) ;
#5949=AXIS2_PLACEMENT_3D ( 'NONE', #350, #22407, #524 ) ;
#5956=DIRECTION ( 'NONE',  ( -1.000000000000000000, 0.000000000000000000, 0.000000000000000000 ) ) ;
#5986=DIRECTION ( 'NONE',  ( -1.000000000000000000, 0.000000000000000000, 0.000000000000000000 ) ) ;
#6000=VECTOR ( 'NONE', #441, 1000.000000000000000 ) ;
#6005=CARTESIAN_POINT ( 'NONE',  ( -108.1236054928398573, -4.063426306576022995, 6.307665442424295499 ) ) ;
#6015=ORIENTED_EDGE ( 'NONE', *, *, #13544, .T. ) ;
#6035=CARTESIAN_POINT ( 'NONE',  ( -105.6811520247811558, -5.080615126163384510, 11.42114788619747046 ) ) ;
#6040=VERTEX_POINT ( 'NONE', #15323 ) ;
#6050=CARTESIAN_POINT ( 'NONE',  ( -109.9479883445679178, -1.339152422118500718, -12.43243648734289408 ) ) ;
#6053=DIRECTION ( 'NONE',  ( -0.000000000000000000, -0.000000000000000000, -1.000000000000000000 ) ) ;
#6057=EDGE_CURVE ( 'NONE', #23099, #30505, #25986, .T. ) ;
#6075=AXIS2_PLACEMENT_3D ( 'NONE', #5188, #26915, #13408 ) ;
#6092=ORIENTED_EDGE ( 'NONE', *, *, #29545, .T. ) ;
#6105=CARTESIAN_POINT ( 'NONE',  ( 107.8902921054316124, -4.970825052104117070, -11.47130252761374081 ) ) ;
#6116=CARTESIAN_POINT ( 'NONE',  ( 99.26191511054632599, -4.118294838564020743E-16, -7.500000000000000000 ) ) ;
#6159=ORIENTED_EDGE ( 'NONE', *, *, #26308, .F. ) ;
#6184=ORIENTED_EDGE ( 'NONE', *, *, #9000, .F. ) ;
#6202=VERTEX_POINT ( 'NONE', #32369 ) ;
#6220=FACE_OUTER_BOUND ( 'NONE', #19856, .T. ) ;
#6286=PLANE ( 'NONE',  #30301 ) ;
#6326=ADVANCED_FACE ( 'NONE', ( #11560 ), #25056, .T. ) ;
#6342=CARTESIAN_POINT ( 'NONE',  ( -101.1521832138544994, 3.386225727737903313, 12.03506400121763065 ) ) ;
#6362=ORIENTED_EDGE ( 'NONE', *, *, #11901, .F. ) ;
#6380=CARTESIAN_POINT ( 'NONE',  ( 110.1470437452871920, 2.564129753321950478, 12.23925059504672674 ) ) ;
#6389=CARTESIAN_POINT ( 'NONE',  ( -103.6615931442450602, -4.948512067686756666, 11.47900473831605161 ) ) ;
#6425=EDGE_CURVE ( 'NONE', #22922, #16360, #9752, .T. ) ;
#6459=FACE_BOUND ( 'NONE', #25958, .T. ) ;
#6472=CARTESIAN_POINT ( 'NONE',  ( 102.0984371113816991, 4.963291960430601613, -5.628698742319545367 ) ) ;
#6505=CARTESIAN_POINT ( 'NONE',  ( -130.6469666100234406, 6.000000000000000000, 57.49999999999999289 ) ) ;
#6554=ORIENTED_EDGE ( 'NONE', *, *, #1990, .F. ) ;
#6566=CARTESIAN_POINT ( 'NONE',  ( -99.88497961182919482, 6.264410040187948829E-16, -12.50000000000000000 ) ) ;
#6570=CARTESIAN_POINT ( 'NONE',  ( -108.8497219713561179, -3.384384043357604899, 12.03563115889556201 ) ) ;
#6585=CARTESIAN_POINT ( 'NONE',  ( -108.3801912069810101, -3.853301823223607592, -11.89378582241139171 ) ) ;
#6620=DIRECTION ( 'NONE',  ( -1.000000000000000000, 0.000000000000000000, 0.000000000000000000 ) ) ;
#6643=VERTEX_POINT ( 'NONE', #23808 ) ;
#6647=CARTESIAN_POINT ( 'NONE',  ( 102.4136796593249130, 5.135442232304142429, -5.469792608531489186 ) ) ;
#6712=CARTESIAN_POINT ( 'NONE',  ( 127.4999999999999147, 0.000000000000000000, 0.000000000000000000 ) ) ;
#6731=CARTESIAN_POINT ( 'NONE',  ( 109.5450345215125196, 3.507529710008592705, 11.99873639479134546 ) ) ;
#6736=AXIS2_PLACEMENT_3D ( 'NONE', #8916, #33118, #8734 ) ;
#6745=CARTESIAN_POINT ( 'NONE',  ( -101.1547991473559449, -3.377194313163046857, 12.03587146382073847 ) ) ;
#6761=CARTESIAN_POINT ( 'NONE',  ( -106.3384068557549256, -4.948512067686755778, -11.47900473831604806 ) ) ;
#6764=DIRECTION ( 'NONE',  ( -1.000000000000000000, -0.000000000000000000, -0.000000000000000000 ) ) ;
#6765=ORIENTED_EDGE ( 'NONE', *, *, #24038, .F. ) ;
#6792=VECTOR ( 'NONE', #30176, 1000.000000000000000 ) ;
#6834=CARTESIAN_POINT ( 'NONE',  ( 109.5174362172994620, -3.557362730766958858, -6.611294427798556583 ) ) ;
#6983=CARTESIAN_POINT ( 'NONE',  ( -130.6469666100234406, -6.000000000000000000, 62.49999999999999289 ) ) ;
#6995=CARTESIAN_POINT ( 'NONE',  ( 110.5282433365937607, 1.549642152983123244, -7.340597171393927312 ) ) ;
#6997=CARTESIAN_POINT ( 'NONE',  ( -103.6344077460457385, 4.941456866685308036, -5.642756420309244625 ) ) ;
#7001=CARTESIAN_POINT ( 'NONE',  ( 110.5497257000961042, 1.507575458593801265, -12.41447922803858894 ) ) ;
#7043=ORIENTED_EDGE ( 'NONE', *, *, #2471, .T. ) ;
#7055=CARTESIAN_POINT ( 'NONE',  ( 99.30043414807218483, -0.7644170489479770181, 12.48218521077886400 ) ) ;
#7130=LINE ( 'NONE', #18027, #28595 ) ;
#7135=EDGE_CURVE ( 'NONE', #3925, #13528, #21619, .T. ) ;
#7136=EDGE_CURVE ( 'NONE', #13528, #26514, #5225, .T. ) ;
#7139=VERTEX_POINT ( 'NONE', #17009 ) ;
#7146=ORIENTED_EDGE ( 'NONE', *, *, #10323, .F. ) ;
#7171=CARTESIAN_POINT ( 'NONE',  ( 100.4549654784875088, 3.507529710008591373, -11.99873639479134368 ) ) ;
#7215=CARTESIAN_POINT ( 'NONE',  ( -110.1150203881707910, 0.3368795255050305859, 12.50000000000000178 ) ) ;
#7232=CARTESIAN_POINT ( 'NONE',  ( -110.1150203881707910, 3.829664765295703645E-16, -7.500000000000000000 ) ) ;
#7271=CARTESIAN_POINT ( 'NONE',  ( 99.46260833598724105, -1.553728400065965687, 7.347407880389961399 ) ) ;
#7301=CARTESIAN_POINT ( 'NONE',  ( -130.6469666100234406, 6.000000000000000000, -57.49999999999999289 ) ) ;
#7304=VECTOR ( 'NONE', #11879, 1000.000000000000000 ) ;
#7337=CARTESIAN_POINT ( 'NONE',  ( 108.7790296513208119, 4.332787265952012135, -6.129206022554251732 ) ) ;
#7344=CARTESIAN_POINT ( 'NONE',  ( 108.7969789446760132, 4.317991217963451867, -11.73376546078468508 ) ) ;
#7345=( NAMED_UNIT ( * ) PLANE_ANGLE_UNIT ( ) SI_UNIT ( $, .RADIAN. ) );
#7398=CARTESIAN_POINT ( 'NONE',  ( 100.3426091166337812, -3.356891575080633849, 12.04186941445821724 ) ) ;
#7417=DIRECTION ( 'NONE',  ( 0.000000000000000000, -0.000000000000000000, -1.000000000000000000 ) ) ;
#7447=CARTESIAN_POINT ( 'NONE',  ( 104.8054821786513884, -5.738162003225207641, 4.829440634198706839 ) ) ;
#7457=CIRCLE ( 'NONE', #5170, 7.500000000000000000 ) ;
#7487=EDGE_CURVE ( 'NONE', #12045, #11373, #29420, .T. ) ;
#7516=CARTESIAN_POINT ( 'NONE',  ( -109.0419893062853305, 3.151985035376887456, -6.811940677030117186 ) ) ;
#7519=CARTESIAN_POINT ( 'NONE',  ( 102.9575692563913236, 5.365524250098477665, -11.29014866489559843 ) ) ;
#7546=DIRECTION ( 'NONE',  ( -0.000000000000000000, 0.000000000000000000, 1.000000000000000000 ) ) ;
#7580=CARTESIAN_POINT ( 'NONE',  ( -100.4342740665978084, -2.311989032590066717, -7.136426621730634245 ) ) ;
#7581=CARTESIAN_POINT ( 'NONE',  ( 212.5000000000000000, 1.224646799147353256E-15, -10.00000000000000000 ) ) ;
#7583=EDGE_LOOP ( 'NONE', ( #22541, #13466, #20401, #12866 ) ) ;
#7605=CARTESIAN_POINT ( 'NONE',  ( -105.6755875751734948, 5.081434799294424209, -11.42078282599713468 ) ) ;
#7629=CARTESIAN_POINT ( 'NONE',  ( 105.9811049962103056, -5.656875047978680904, 4.924762495648698390 ) ) ;
#7646=ORIENTED_EDGE ( 'NONE', *, *, #7136, .F. ) ;
#7652=ADVANCED_FACE ( 'NONE', ( #16610 ), #30471, .T. ) ;
#7657=DIRECTION ( 'NONE',  ( 1.000000000000000000, 0.000000000000000000, 0.000000000000000000 ) ) ;
#7676=CARTESIAN_POINT ( 'NONE',  ( 127.4999999999999147, 0.000000000000000000, 0.000000000000000000 ) ) ;
#7696=CARTESIAN_POINT ( 'NONE',  ( 109.9315740078916690, 2.939425563888521609, -6.902236325305502795 ) ) ;
#7705=CARTESIAN_POINT ( 'NONE',  ( 110.7008314884919287, 0.7568087271434544849, -12.48276086518024464 ) ) ;
#7711=VECTOR ( 'NONE', #29628, 1000.000000000000000 ) ;
#7716=VERTEX_POINT ( 'NONE', #32776 ) ;
#7719=CARTESIAN_POINT ( 'NONE',  ( 110.7380848894536598, 7.027127293105237708E-16, -57.49999999999999289 ) ) ;
#7729=VECTOR ( 'NONE', #1309, 1000.000000000000000 ) ;
#7758=CARTESIAN_POINT ( 'NONE',  ( -99.88497961182923746, 0.3508469386294337244, 7.500000000000000888 ) ) ;
#7762=CARTESIAN_POINT ( 'NONE',  ( -103.6349267833586651, -4.941537997685731654, -5.642681918066577929 ) ) ;
#7768=B_SPLINE_CURVE_WITH_KNOTS ( 'NONE', 3,
 ( #8083, #19140, #11123, #14143, #27654, #21785, #32811, #5742, #30511, #13609, #781, #16469, #3091, #14325, #25152, #6105, #21616, #30144, #257, #32456, #32980, #21970, #24973, #8437, #27828, #19310, #16646, #8605, #18958, #19666, #5927, #29801, #27479, #17004, #5406, #604, #29978, #32633, #5573, #11294, #16294, #27126, #8260 ),
 .UNSPECIFIED., .F., .F.,
 ( 4, 2, 2, 2, 2, 2, 2, 2, 2, 2, 2, 1, 2, 2, 2, 2, 2, 2, 2, 2, 2, 4 ),
 ( 0.01819865299508306028, 0.01933465672311146522, 0.02047066045113987015, 0.02103866231515406568, 0.02160666417916826121, 0.02217466604318245327, 0.02274266790719664880, 0.02387867163522501210, 0.02501467536325337540, 0.02615067909128173870, 0.02671868095529592035, 0.02728668281931010547, 0.02785468468332428366, 0.02842268654733846878, 0.02955869027536687371, 0.03069469400339527518, 0.03183069773142367664, 0.03296670145945208852, 0.03353470332346628752, 0.03410270518748048652, 0.03523870891550889839, 0.03637471264353730332 ),
 .UNSPECIFIED. ) ;
#7775=FACE_OUTER_BOUND ( 'NONE', #31395, .T. ) ;
#7789=EDGE_CURVE ( 'NONE', #6643, #2811, #34451, .T. ) ;
#7805=CIRCLE ( 'NONE', #17508, 10.00000000000000000 ) ;
#7806=DIRECTION ( 'NONE',  ( -0.000000000000000000, -0.000000000000000000, -1.000000000000000000 ) ) ;
#7845=DIRECTION ( 'NONE',  ( -1.000000000000000000, 0.000000000000000000, 0.000000000000000000 ) ) ;
#7870=ORIENTED_EDGE ( 'NONE', *, *, #13875, .F. ) ;
#7881=CARTESIAN_POINT ( 'NONE',  ( -100.1623731062489355, 1.695881020439946596, -7.312931660397135047 ) ) ;
#7884=ORIENTED_EDGE ( 'NONE', *, *, #175, .T. ) ;
#7890=CARTESIAN_POINT ( 'NONE',  ( -110.1150203881707910, 3.829664765295703645E-16, -7.500000000000000000 ) ) ;
#7911=CYLINDRICAL_SURFACE ( 'NONE', #10843, 5.738084889453667792 ) ;
#7935=CARTESIAN_POINT ( 'NONE',  ( -102.4133971961325926, 4.424631548980197060, 6.059743929710633026 ) ) ;
#7942=CARTESIAN_POINT ( 'NONE',  ( -100.5942677908518306, -2.603972021169325135, -7.035140931575556422 ) ) ;
#7961=DIRECTION ( 'NONE',  ( -1.000000000000000000, 0.000000000000000000, 0.000000000000000000 ) ) ;
#7963=CARTESIAN_POINT ( 'NONE',  ( -101.1480816615366223, 3.381649300054700991, -12.03636906590512723 ) ) ;
#7975=CARTESIAN_POINT ( 'NONE',  ( 212.5000000000000000, 0.000000000000000000, 7.500000000000000000 ) ) ;
#7979=CARTESIAN_POINT ( 'NONE',  ( -110.0447977791740897, -0.8621751556914719616, 7.452240479933210260 ) ) ;
#8021=CARTESIAN_POINT ( 'NONE',  ( 100.0684259921083452, 2.939425563888521609, 6.902236325305502795 ) ) ;
#8058=CARTESIAN_POINT ( 'NONE',  ( 110.6566244370989551, -0.9828571727418841109, -7.437816238889399578 ) ) ;
#8076=AXIS2_PLACEMENT_3D ( 'NONE', #34990, #32296, #29634 ) ;
#8083=CARTESIAN_POINT ( 'NONE',  ( 110.7380848894536598, 7.027143731242819742E-16, -12.50000000000000000 ) ) ;
#8093=ORIENTED_EDGE ( 'NONE', *, *, #7487, .T. ) ;
#8111=CARTESIAN_POINT ( 'NONE',  ( -108.1240957144767521, 4.062957613056745743, 6.307943406627045668 ) ) ;
#8139=CARTESIAN_POINT ( 'NONE',  ( -109.4325559004959416, 2.574279381791157562, -12.23535145228420085 ) ) ;
#8158=CARTESIAN_POINT ( 'NONE',  ( -105.6898066376448497, -5.079998963781828358, 5.518357322521167951 ) ) ;
#8160=ORIENTED_EDGE ( 'NONE', *, *, #2272, .F. ) ;
#8200=CARTESIAN_POINT ( 'NONE',  ( 99.47175666340625355, 1.549642152983123244, 7.340597171393927312 ) ) ;
#8201=PRODUCT_CONTEXT ( 'NONE', #29861, 'mechanical' ) ;
#8212=CARTESIAN_POINT ( 'NONE',  ( 0.000000000000000000, 0.000000000000000000, 62.49999999999999289 ) ) ;
#8260=CARTESIAN_POINT ( 'NONE',  ( 99.26191511054632599, -6.978196330887525654E-16, -12.50000000000000000 ) ) ;
#8267=VERTEX_POINT ( 'NONE', #17414 ) ;
#8273=ORIENTED_EDGE ( 'NONE', *, *, #2585, .T. ) ;
#8289=ORIENTED_EDGE ( 'NONE', *, *, #27121, .T. ) ;
#8291=CARTESIAN_POINT ( 'NONE',  ( -109.4378652105823306, 2.632420417224709652, 7.052679658646592742 ) ) ;
#8310=CARTESIAN_POINT ( 'NONE',  ( 119.9999999999998295, 0.000000000000000000, 0.000000000000000000 ) ) ;
#8336=AXIS2_PLACEMENT_3D ( 'NONE', #28207, #25351, #22703 ) ;
#8341=CARTESIAN_POINT ( 'NONE',  ( -101.2785545903827824, -3.512874579320472535, 6.627714125729965211 ) ) ;
#8374=VECTOR ( 'NONE', #12146, 1000.000000000000000 ) ;
#8381=CARTESIAN_POINT ( 'NONE',  ( 102.9210534578009657, 5.351410369513340370, 5.255735268165820706 ) ) ;
#8392=ORIENTED_EDGE ( 'NONE', *, *, #25680, .F. ) ;
#8416=CARTESIAN_POINT ( 'NONE',  ( 110.1177974931836303, -2.622468385745837072, -7.036045090041716854 ) ) ;
#8419=ORIENTED_EDGE ( 'NONE', *, *, #31180, .T. ) ;
#8429=CARTESIAN_POINT ( 'NONE',  ( -105.0000000000000000, 0.000000000000000000, 60.00000000000000000 ) ) ;
#8433=CARTESIAN_POINT ( 'NONE',  ( 127.4999999999999147, 1.530808498934191521E-15, -12.50000000000000000 ) ) ;
#8437=CARTESIAN_POINT ( 'NONE',  ( 104.6251203501937113, -5.728975534391925528, -11.10987307012756276 ) ) ;
#8474=DIRECTION ( 'NONE',  ( 1.000000000000000000, -0.000000000000000000, -0.000000000000000000 ) ) ;
#8498=CARTESIAN_POINT ( 'NONE',  ( -100.5674440995040442, 2.574279381791158450, 12.23535145228419907 ) ) ;
#8516=CARTESIAN_POINT ( 'NONE',  ( -104.1337689642702600, -5.044029065977395199, 5.550668370081901948 ) ) ;
#8543=EDGE_CURVE ( 'NONE', #12316, #14561, #8614, .T. ) ;
#8570=ORIENTED_EDGE ( 'NONE', *, *, #23719, .T. ) ;
#8579=ORIENTED_EDGE ( 'NONE', *, *, #29645, .F. ) ;
#8598=VERTEX_POINT ( 'NONE', #31216 ) ;
#8605=CARTESIAN_POINT ( 'NONE',  ( 103.1365178746234363, -5.440007577125886229, -11.25529792293082032 ) ) ;
#8614=LINE ( 'NONE', #3443, #29857 ) ;
#8635=EDGE_CURVE ( 'NONE', #19142, #13351, #3968, .T. ) ;
#8656=ORIENTED_EDGE ( 'NONE', *, *, #13626, .T. ) ;
#8692=DIRECTION ( 'NONE',  ( 0.000000000000000000, 0.000000000000000000, -1.000000000000000000 ) ) ;
#8722=EDGE_CURVE ( 'NONE', #30104, #7716, #15917, .T. ) ;
#8731=CARTESIAN_POINT ( 'NONE',  ( -103.3404196479744570, -4.849832969747407851, -11.52164913186504513 ) ) ;
#8734=DIRECTION ( 'NONE',  ( 0.000000000000000000, 0.000000000000000000, 1.000000000000000000 ) ) ;
#8767=ORIENTED_EDGE ( 'NONE', *, *, #33879, .T. ) ;
#8791=EDGE_CURVE ( 'NONE', #549, #18500, #2352, .T. ) ;
#8813=VECTOR ( 'NONE', #15130, 1000.000000000000000 ) ;
#8815=CARTESIAN_POINT ( 'NONE',  ( 103.0960974094320903, -5.425683864377651489, -5.182047996533464485 ) ) ;
#8851=ADVANCED_FACE ( 'NONE', ( #18401 ), #4844, .T. ) ;
#8853=ORIENTED_EDGE ( 'NONE', *, *, #3678, .F. ) ;
#8881=EDGE_CURVE ( 'NONE', #12045, #26496, #14290, .T. ) ;
#8888=EDGE_CURVE ( 'NONE', #2593, #22922, #7805, .T. ) ;
#8916=CARTESIAN_POINT ( 'NONE',  ( 119.9999999999998295, 0.000000000000000000, 0.000000000000000000 ) ) ;
#8980=FACE_OUTER_BOUND ( 'NONE', #14185, .T. ) ;
#9000=EDGE_CURVE ( 'NONE', #14417, #16671, #14815, .T. ) ;
#9018=AXIS2_PLACEMENT_3D ( 'NONE', #6712, #4384, #25580 ) ;
#9070=FACE_OUTER_BOUND ( 'NONE', #33542, .T. ) ;
#9074=CARTESIAN_POINT ( 'NONE',  ( -107.5741775841794095, -4.432411119407283273, 11.68939833797860395 ) ) ;
#9100=DIRECTION ( 'NONE',  ( 0.000000000000000000, -1.000000000000000000, 0.000000000000000000 ) ) ;
#9149=CARTESIAN_POINT ( 'NONE',  ( 101.5050109452463403, 4.564908081027950537, -5.956352141036524550 ) ) ;
#9152=VECTOR ( 'NONE', #16962, 1000.000000000000000 ) ;
#9210=DIRECTION ( 'NONE',  ( -1.000000000000000000, 0.000000000000000000, 0.000000000000000000 ) ) ;
#9219=CARTESIAN_POINT ( 'NONE',  ( -130.6469666100234406, 6.000000000000000000, -62.49999999999999289 ) ) ;
#9245=CARTESIAN_POINT ( 'NONE',  ( -130.6469666100234406, -6.000000000000000000, -62.49999999999999289 ) ) ;
#9251=CARTESIAN_POINT ( 'NONE',  ( -109.0610159990791175, -3.127506413740516411, 12.10571963949989005 ) ) ;
#9253=DIRECTION ( 'NONE',  ( 0.000000000000000000, -1.000000000000000000, 0.000000000000000000 ) ) ;
#9259=VECTOR ( 'NONE', #13102, 1000.000000000000000 ) ;
#9260=ORIENTED_EDGE ( 'NONE', *, *, #27993, .T. ) ;
#9266=CARTESIAN_POINT ( 'NONE',  ( -100.0523001014507827, -1.340877102867427562, -12.43231962408541769 ) ) ;
#9268=AXIS2_PLACEMENT_3D ( 'NONE', #26741, #23550, #1663 ) ;
#9285=B_SPLINE_CURVE_WITH_KNOTS ( 'NONE', 3,
 ( #24351, #32719, #21864, #5482, #7979, #27732, #13863, #156, #5304, #27555, #21687, #4253, #32536, #11371, #6005, #18863, #30060, #5827, #24702, #8158, #13683, #3171, #27377, #2816, #8516, #11198, #341, #13350, #16197, #27206, #19384, #8341, #30224, #16723, #14042, #24879, #10676, #19043, #22222, #11015, #2648, #29885, #5650, #33063 ),
 .UNSPECIFIED., .F., .F.,
 ( 4, 2, 2, 2, 2, 2, 2, 2, 2, 2, 2, 2, 2, 2, 2, 2, 2, 2, 2, 2, 2, 4 ),
 ( 0.01657113979051928407, 0.01708818281900468042, 0.01760522584749007330, 0.01863931190446085559, 0.01915635493294623806, 0.01967339796143162400, 0.02070748401840238895, 0.02174157007537315736, 0.02277565613234392577, 0.02380974218931469419, 0.02484382824628546260, 0.02536087127477082426, 0.02587791430325619285, 0.02691200036022687453, 0.02794608641719755968, 0.02898017247416824482, 0.02949721550265357872, 0.03001425853113890568, 0.03104834458810954573, 0.03156538761659487269, 0.03208243064508019965, 0.03311651670205084663 ),
 .UNSPECIFIED. ) ;
#9287=CARTESIAN_POINT ( 'NONE',  ( 212.5000000000000000, 1.224646799147353256E-15, -10.00000000000000000 ) ) ;
#9297=DIRECTION ( 'NONE',  ( -0.000000000000000000, -0.000000000000000000, -1.000000000000000000 ) ) ;
#9308=EDGE_LOOP ( 'NONE', ( #33651, #23780 ) ) ;
#9333=CARTESIAN_POINT ( 'NONE',  ( -117.4999999999997442, 1.530808498934191521E-15, -12.50000000000000000 ) ) ;
#9336=EDGE_CURVE ( 'NONE', #34071, #17516, #19068, .T. ) ;
#9393=AXIS2_PLACEMENT_3D ( 'NONE', #28469, #34684, #12981 ) ;
#9426=CARTESIAN_POINT ( 'NONE',  ( 104.0527614346196970, 5.662516510817761528, 11.14395138485681791 ) ) ;
#9435=CARTESIAN_POINT ( 'NONE',  ( -110.1150203881707910, 3.166944581793445397E-20, 12.50000000000000000 ) ) ;
#9446=ADVANCED_FACE ( 'NONE', ( #9070 ), #11757, .T. ) ;
#9454=CARTESIAN_POINT ( 'NONE',  ( -101.1502780286438679, -3.384384043357604011, -12.03563115889556379 ) ) ;
#9458=VERTEX_POINT ( 'NONE', #6566 ) ;
#9464=DIRECTION ( 'NONE',  ( -0.000000000000000000, -0.000000000000000000, -1.000000000000000000 ) ) ;
#9504=ORIENTED_EDGE ( 'NONE', *, *, #9000, .T. ) ;
#9530=CARTESIAN_POINT ( 'NONE',  ( 102.0964664041139542, -4.962105133902832144, -5.629733210525461828 ) ) ;
#9576=LINE ( 'NONE', #15275, #4443 ) ;
#9595=CARTESIAN_POINT ( 'NONE',  ( 106.3182022809973546, 5.587831648195837886, 11.18158713856774966 ) ) ;
#9642=APPLICATION_CONTEXT ( 'automotive_design' ) ;
#9686=EDGE_LOOP ( 'NONE', ( #32033, #1867, #946, #380, #23424, #8656, #11856, #13878, #6554, #7884, #7646, #21099 ) ) ;
#9704=LINE ( 'NONE', #22727, #18725 ) ;
#9732=ORIENTED_EDGE ( 'NONE', *, *, #31314, .T. ) ;
#9736=AXIS2_PLACEMENT_3D ( 'NONE', #4021, #17599, #4539 ) ;
#9752=LINE ( 'NONE', #1221, #22440 ) ;
#9756=VERTEX_POINT ( 'NONE', #11404 ) ;
#9758=CARTESIAN_POINT ( 'NONE',  ( 110.4374853395854643, 1.870982065537967420, 12.36420004006153839 ) ) ;
#9783=CARTESIAN_POINT ( 'NONE',  ( 107.9035335958860173, -4.962105133902832144, 5.629733210525461828 ) ) ;
#9810=ADVANCED_FACE ( 'NONE', ( #6220, #14794 ), #17115, .T. ) ;
#9819=CARTESIAN_POINT ( 'NONE',  ( 0.000000000000000000, 0.000000000000000000, -62.49999999999999289 ) ) ;
#9822=ORIENTED_EDGE ( 'NONE', *, *, #13916, .F. ) ;
#9834=VECTOR ( 'NONE', #27095, 1000.000000000000000 ) ;
#9848=CARTESIAN_POINT ( 'NONE',  ( 110.7380848894539866, -2.712459438615764475E-14, -7.500000000000241585 ) ) ;
#9850=CARTESIAN_POINT ( 'NONE',  ( -110.1150203881708194, 0.3508469386294343906, -7.500000000000001776 ) ) ;
#9854=CARTESIAN_POINT ( 'NONE',  ( 99.26191511054634020, 0.3849557905273010561, -12.50000000000000533 ) ) ;
#9868=ORIENTED_EDGE ( 'NONE', *, *, #2272, .T. ) ;
#9875=DIRECTION ( 'NONE',  ( -0.000000000000000000, -0.000000000000000000, 1.000000000000000000 ) ) ;
#9913=CARTESIAN_POINT ( 'NONE',  ( 104.9965108525136372, -5.747432480335291416, 11.10030588989970468 ) ) ;
#9920=CARTESIAN_POINT ( 'NONE',  ( -110.0792196684870987, -0.6954373895739790479, -7.475453221064620735 ) ) ;
#9928=FACE_OUTER_BOUND ( 'NONE', #9686, .T. ) ;
#9939=AXIS2_PLACEMENT_3D ( 'NONE', #8212, #2521, #32771 ) ;
#9943=LINE ( 'NONE', #18157, #30876 ) ;
#9948=DIRECTION ( 'NONE',  ( -1.000000000000000000, 0.000000000000000000, 0.000000000000000000 ) ) ;
#9960=CARTESIAN_POINT ( 'NONE',  ( 109.9257156030288911, -2.949151772667967020, 6.898053038626237310 ) ) ;
#9977=VECTOR ( 'NONE', #22724, 1000.000000000000000 ) ;
#9987=DIRECTION ( 'NONE',  ( -0.000000000000000000, -0.000000000000000000, 1.000000000000000000 ) ) ;
#10026=CARTESIAN_POINT ( 'NONE',  ( 106.5416737992720755, 5.530333585247596773, -5.066783516361279993 ) ) ;
#10032=CARTESIAN_POINT ( 'NONE',  ( 101.2072798900310175, 4.321688686550378300, -11.73238900788529904 ) ) ;
#10059=DIRECTION ( 'NONE',  ( -1.000000000000000000, 0.000000000000000000, 0.000000000000000000 ) ) ;
#10080=AXIS2_PLACEMENT_3D ( 'NONE', #8310, #5273, #32334 ) ;
#10089=CARTESIAN_POINT ( 'NONE',  ( 110.1379535922845463, -2.561659524636492602, 12.23586498300001679 ) ) ;
#10094=CARTESIAN_POINT ( 'NONE',  ( -104.3101933623550792, -5.079998963781827470, -5.518357322521168840 ) ) ;
#10107=DIRECTION ( 'NONE',  ( 0.000000000000000000, -1.000000000000000000, 0.000000000000000000 ) ) ;
#10110=CARTESIAN_POINT ( 'NONE',  ( 99.29916851150809975, 0.7568087271434508212, 12.48276086518024641 ) ) ;
#10123=PLANE ( 'NONE',  #9393 ) ;
#10136=CARTESIAN_POINT ( 'NONE',  ( 99.26191511054601335, -2.804307960831458189E-14, 7.500000000000241585 ) ) ;
#10145=EDGE_LOOP ( 'NONE', ( #12310, #15522, #4076, #2166 ) ) ;
#10151=CIRCLE ( 'NONE', #13014, 10.00000000000000000 ) ;
#10208=CARTESIAN_POINT ( 'NONE',  ( 107.8898084714338523, 4.971174042719110453, -11.47116230092015066 ) ) ;
#10220=VERTEX_POINT ( 'NONE', #25406 ) ;
#10237=ADVANCED_FACE ( 'NONE', ( #1387 ), #19854, .T. ) ;
#10246=CARTESIAN_POINT ( 'NONE',  ( 129.3530333899765594, 6.000000000000000000, -62.49999999999999289 ) ) ;
#10253=EDGE_CURVE ( 'NONE', #31150, #26496, #9576, .T. ) ;
#10270=ORIENTED_EDGE ( 'NONE', *, *, #13618, .F. ) ;
#10273=B_SPLINE_CURVE_WITH_KNOTS ( 'NONE', 3,
 ( #9435, #31146, #25077, #28300, #896, #22780, #17104, #3894, #22612, #33454, #33629, #9251, #6570, #33096, #11937, #9074, #11582, #27937, #25261, #6035, #715, #4063, #11763, #6389, #20119, #28116, #16932, #14435, #25439, #3729, #6745, #30965, #17287, #25791, #25612, #19769, #19940, #30788, #3375, #17470 ),
 .UNSPECIFIED., .F., .F.,
 ( 4, 2, 2, 2, 2, 2, 2, 2, 2, 2, 2, 2, 2, 2, 2, 2, 2, 2, 2, 4 ),
 ( 0.01617148595533309322, 0.01667647242675793923, 0.01718145889818278524, 0.01819143184103248073, 0.01869641831245732674, 0.01920140478388217276, 0.02021137772673184396, 0.02122135066958151517, 0.02223132361243118638, 0.02324129655528085758, 0.02425126949813052879, 0.02526124244098020000, 0.02627121538382987120, 0.02728118832667954241, 0.02829116126952921362, 0.02879614774095406310, 0.02930113421237891258, 0.03031110715522861154, 0.03132108009807831051, 0.03233105304092800947 ),
 .UNSPECIFIED. ) ;
#10322=AXIS2_PLACEMENT_3D ( 'NONE', #5075, #32661, #2243 ) ;
#10323=EDGE_CURVE ( 'NONE', #14417, #7139, #10151, .T. ) ;
#10349=ORIENTED_EDGE ( 'NONE', *, *, #17479, .F. ) ;
#10361=CLOSED_SHELL ( 'NONE', ( #9446, #376, #3253, #15406, #24092, #18099, #58, #30733, #3038, #16366, #13200, #31367, #21586, #2156, #6326, #8851, #15656, #15369, #16651, #9810, #31269, #10237, #1255, #7652, #4622, #4239, #3852, #27622, #12640, #13749, #16504, #14399, #28170, #22336, #20493, #4721, #17402, #16411 ) ) ;
#10367=ORIENTED_EDGE ( 'NONE', *, *, #2037, .T. ) ;
#10377=CARTESIAN_POINT ( 'NONE',  ( 109.2888833233461980, 3.828784459365716319, -6.456053091683092049 ) ) ;
#10433=B_SPLINE_CURVE_WITH_KNOTS ( 'NONE', 3,
 ( #23957, #32321, #15809, #12956, #5089, #15976, #26639, #4731, #7580, #7942, #13469, #12782, #2252, #23626, #15627, #34838, #5258, #31626, #7762, #10094, #10629, #18818, #34657, #10448, #2422, #18481, #13122, #2600, #13305, #32154, #18649, #29495, #29663, #26813, #16151, #24134, #35016, #21481, #4910, #26994, #24307, #9920, #20780, #7232 ),
 .UNSPECIFIED., .F., .F.,
 ( 4, 2, 2, 2, 2, 2, 2, 2, 2, 2, 2, 2, 2, 2, 2, 2, 2, 2, 2, 2, 2, 4 ),
 ( 0.01657113979051930489, 0.01708818281900469430, 0.01760522584749008371, 0.01863931190446085212, 0.01915635493294623806, 0.01967339796143162400, 0.02070748401840239589, 0.02174157007537316777, 0.02277565613234393965, 0.02380974218931471154, 0.02484382824628548342, 0.02536087127477085201, 0.02587791430325621367, 0.02691200036022690575, 0.02794608641719759437, 0.02898017247416828646, 0.02949721550265361689, 0.03001425853113894732, 0.03104834458810958736, 0.03156538761659492126, 0.03208243064508024822, 0.03311651670205089520 ),
 .UNSPECIFIED. ) ;
#10448=CARTESIAN_POINT ( 'NONE',  ( -105.6966460872811524, -5.070312235224274211, -5.526528498279826174 ) ) ;
#10539=CARTESIAN_POINT ( 'NONE',  ( 109.2869635376109443, 3.831042253767035444, 6.454752727393734624 ) ) ;
#10561=CARTESIAN_POINT ( 'NONE',  ( 127.4999999999999147, 1.530808498934191521E-15, -12.50000000000000000 ) ) ;
#10569=CARTESIAN_POINT ( 'NONE',  ( 106.8659954277186586, 5.439315735761661941, -11.25565174199232743 ) ) ;
#10626=CARTESIAN_POINT ( 'NONE',  ( -103.6327063011913623, 4.940661300061107042, 5.643441299694565316 ) ) ;
#10628=DIRECTION ( 'NONE',  ( 0.000000000000000000, 0.000000000000000000, -1.000000000000000000 ) ) ;
#10629=CARTESIAN_POINT ( 'NONE',  ( -104.6531427807880306, -5.115148824049938092, -5.485002510375801776 ) ) ;
#10653=CARTESIAN_POINT ( 'NONE',  ( -104.3222861221629358, 5.081071289440265204, -11.42094332255972766 ) ) ;
#10676=CARTESIAN_POINT ( 'NONE',  ( -100.4263556498910646, -2.314419832420931744, 7.141071956987316227 ) ) ;
#10715=VECTOR ( 'NONE', #6053, 1000.000000000000000 ) ;
#10718=EDGE_LOOP ( 'NONE', ( #9822, #12513, #15546, #22496 ) ) ;
#10773=CARTESIAN_POINT ( 'NONE',  ( 212.5000000000000000, 9.184850993605147944E-16, -7.500000000000000000 ) ) ;
#10795=CARTESIAN_POINT ( 'NONE',  ( -106.6861857794938544, 4.840548292904078842, 5.731216124222061836 ) ) ;
#10798=DIRECTION ( 'NONE',  ( -1.000000000000000000, -0.000000000000000000, -0.000000000000000000 ) ) ;
#10802=CARTESIAN_POINT ( 'NONE',  ( 110.7380848894539866, -2.712459438615764475E-14, -7.500000000000241585 ) ) ;
#10843=AXIS2_PLACEMENT_3D ( 'NONE', #18785, #29626, #5223 ) ;
#10853=EDGE_CURVE ( 'NONE', #9458, #10220, #29198, .T. ) ;
#10905=CARTESIAN_POINT ( 'NONE',  ( -119.9999999999997726, 0.000000000000000000, 0.000000000000000000 ) ) ;
#10910=LINE ( 'NONE', #21591, #348 ) ;
#10970=PLANE ( 'NONE',  #13325 ) ;
#11015=CARTESIAN_POINT ( 'NONE',  ( -100.0688062106723919, -1.369675690685149050, 7.375755714855094070 ) ) ;
#11049=ORIENTED_EDGE ( 'NONE', *, *, #14200, .T. ) ;
#11063=CARTESIAN_POINT ( 'NONE',  ( 102.0965294410245576, 4.962255517573300523, 5.629655879752474057 ) ) ;
#11086=DIRECTION ( 'NONE',  ( 0.000000000000000000, 0.000000000000000000, -1.000000000000000000 ) ) ;
#11121=CARTESIAN_POINT ( 'NONE',  ( -99.88497961182919482, 6.264093345946821604E-16, 60.00000000000000000 ) ) ;
#11123=CARTESIAN_POINT ( 'NONE',  ( 110.6995658519277725, -0.7644170489479740205, -12.48218521077886400 ) ) ;
#11144=EDGE_CURVE ( 'NONE', #32910, #32630, #4934, .T. ) ;
#11154=CARTESIAN_POINT ( 'NONE',  ( -100.9580106937146837, 3.151985035376890565, 6.811940677030119851 ) ) ;
#11182=CARTESIAN_POINT ( 'NONE',  ( -103.6623624504978807, 4.939893293632465543, 11.48260997023825425 ) ) ;
#11198=CARTESIAN_POINT ( 'NONE',  ( -103.6321150747602502, -4.940539628404772898, 5.643550520051347164 ) ) ;
#11235=ORIENTED_EDGE ( 'NONE', *, *, #13626, .F. ) ;
#11237=CARTESIAN_POINT ( 'NONE',  ( 100.4793743644694217, 3.553124229080486085, 6.613494096335986505 ) ) ;
#11294=CARTESIAN_POINT ( 'NONE',  ( 99.45139749831538722, -1.510413401456684790, -12.41397948795682993 ) ) ;
#11301=ORIENTED_EDGE ( 'NONE', *, *, #27716, .F. ) ;
#11321=ORIENTED_EDGE ( 'NONE', *, *, #3704, .T. ) ;
#11334=LINE ( 'NONE', #19343, #16337 ) ;
#11371=CARTESIAN_POINT ( 'NONE',  ( -108.3720725006440659, -3.859727759966182781, 6.435874498883202399 ) ) ;
#11373=VERTEX_POINT ( 'NONE', #23963 ) ;
#11404=CARTESIAN_POINT ( 'NONE',  ( 110.7380848894536598, 7.027127293105233764E-16, 12.50000000000000000 ) ) ;
#11406=CARTESIAN_POINT ( 'NONE',  ( 99.42172009583602232, 1.358924363732619600, 7.378408734721662476 ) ) ;
#11411=CARTESIAN_POINT ( 'NONE',  ( -109.4312689855573097, -2.576157761670755164, -12.23490486094944707 ) ) ;
#11477=B_SPLINE_CURVE_WITH_KNOTS ( 'NONE', 3,
 ( #6116, #19852, #30698, #25342, #17018, #14695, #27841, #3447, #14864, #33533, #9149, #6472, #6647, #25698, #12197, #14341, #25519, #17373, #1151, #31561, #28892, #4491, #34763, #32078, #15381, #10026, #12891, #31729, #20537, #18066, #29059, #7337, #10377, #2015, #20882, #7696, #29247, #23375, #1835, #26212, #6995, #23890, #18403, #21232, #9848 ),
 .UNSPECIFIED., .F., .F.,
 ( 4, 2, 2, 2, 2, 2, 2, 2, 2, 2, 1, 2, 2, 2, 2, 2, 2, 2, 2, 2, 2, 2, 4 ),
 ( 3.984693255910324139E-19, 0.001177949164446570477, 0.002355898328893140520, 0.003533847493339711213, 0.004711796657786281907, 0.005889745822232853034, 0.007067694986679424161, 0.007656669568902727506, 0.008245644151126031718, 0.008834618733349335062, 0.009423593315572640142, 0.01001256789779594349, 0.01060154248001924683, 0.01119051706224255191, 0.01177949164446585525, 0.01295744080891246194, 0.01413538997335907210, 0.01531333913780567879, 0.01590231372002897173, 0.01649128830225226466, 0.01708026288447555760, 0.01766923746669885054, 0.01884718663114543988 ),
 .UNSPECIFIED. ) ;
#11537=DIRECTION ( 'NONE',  ( 1.000000000000000000, 0.000000000000000000, 0.000000000000000000 ) ) ;
#11557=DIRECTION ( 'NONE',  ( 1.000000000000000000, -0.000000000000000000, -0.000000000000000000 ) ) ;
#11559=DIRECTION ( 'NONE',  ( -1.000000000000000000, -0.000000000000000000, -0.000000000000000000 ) ) ;
#11560=FACE_OUTER_BOUND ( 'NONE', #29571, .T. ) ;
#11573=ORIENTED_EDGE ( 'NONE', *, *, #28499, .F. ) ;
#11582=CARTESIAN_POINT ( 'NONE',  ( -107.2764268663271281, -4.592708079286354383, 11.62653478258734907 ) ) ;
#11595=CARTESIAN_POINT ( 'NONE',  ( 101.5015052779749425, 4.562308164568303681, 5.958384794357583836 ) ) ;
#11621=EDGE_CURVE ( 'NONE', #3870, #14310, #28828, .T. ) ;
#11623=DIRECTION ( 'NONE',  ( -1.000000000000000000, 0.000000000000000000, 0.000000000000000000 ) ) ;
#11630=PLANE ( 'NONE',  #22110 ) ;
#11649=LINE ( 'NONE', #11121, #4987 ) ;
#11711=CARTESIAN_POINT ( 'NONE',  ( -101.8751819073018225, 4.063332493481115471, 11.82279441766105954 ) ) ;
#11748=CARTESIAN_POINT ( 'NONE',  ( 104.2406003994089616, 5.690832488206158501, 11.12946004024182933 ) ) ;
#11757=CYLINDRICAL_SURFACE ( 'NONE', #30000, 5.115020388170798959 ) ;
#11763=CARTESIAN_POINT ( 'NONE',  ( -104.3285450821986018, -5.082150419746904291, 11.42046709103397895 ) ) ;
#11780=CARTESIAN_POINT ( 'NONE',  ( -102.4258224158205763, -4.432411119407283273, -11.68939833797860395 ) ) ;
#11856=ORIENTED_EDGE ( 'NONE', *, *, #8791, .T. ) ;
#11862=CARTESIAN_POINT ( 'NONE',  ( 106.5437455398453466, -5.539877390153430170, -5.057044031126181061 ) ) ;
#11879=DIRECTION ( 'NONE',  ( 0.000000000000000000, 1.000000000000000000, 0.000000000000000000 ) ) ;
#11890=ORIENTED_EDGE ( 'NONE', *, *, #27850, .T. ) ;
#11892=CARTESIAN_POINT ( 'NONE',  ( -101.6189403138812821, 3.852356953585670318, 11.89405885704113786 ) ) ;
#11898=ORIENTED_EDGE ( 'NONE', *, *, #27850, .F. ) ;
#11901=EDGE_CURVE ( 'NONE', #9458, #3870, #11649, .T. ) ;
#11909=CARTESIAN_POINT ( 'NONE',  ( 99.26191511054632599, -6.978196330887525654E-16, -12.50000000000000000 ) ) ;
#11931=CYLINDRICAL_SURFACE ( 'NONE', #12671, 10.00000000000000000 ) ;
#11937=CARTESIAN_POINT ( 'NONE',  ( -108.1231672730592095, -4.064293880962485339, 11.82242856119474261 ) ) ;
#11940=EDGE_LOOP ( 'NONE', ( #7146, #9504, #4754, #13427 ) ) ;
#11983=EDGE_CURVE ( 'NONE', #32630, #32910, #3850, .T. ) ;
#12018=CIRCLE ( 'NONE', #31331, 10.00000000000000000 ) ;
#12020=CIRCLE ( 'NONE', #31870, 5.115020388170798959 ) ;
#12036=CARTESIAN_POINT ( 'NONE',  ( 99.30430670822994443, -0.7984011589207654636, -7.467432841349395112 ) ) ;
#12045=VERTEX_POINT ( 'NONE', #6983 ) ;
#12066=CARTESIAN_POINT ( 'NONE',  ( -109.8491107295462683, 1.661471846880725911, 12.39299840842996225 ) ) ;
#12074=CARTESIAN_POINT ( 'NONE',  ( 212.5000000000000000, 0.000000000000000000, 0.000000000000000000 ) ) ;
#12083=DIRECTION ( 'NONE',  ( 0.000000000000000000, 0.000000000000000000, -1.000000000000000000 ) ) ;
#12093=DIRECTION ( 'NONE',  ( -1.000000000000000000, -0.000000000000000000, -0.000000000000000000 ) ) ;
#12102=CARTESIAN_POINT ( 'NONE',  ( 104.6215662523440386, 5.728791326347600688, 11.10996872791848844 ) ) ;
#12130=CARTESIAN_POINT ( 'NONE',  ( -109.5893175474791690, -2.283823867687211795, -12.29365298152801778 ) ) ;
#12132=DIRECTION ( 'NONE',  ( -0.000000000000000000, -0.000000000000000000, -1.000000000000000000 ) ) ;
#12133=LINE ( 'NONE', #33831, #21508 ) ;
#12146=DIRECTION ( 'NONE',  ( -1.000000000000000000, -0.000000000000000000, -0.000000000000000000 ) ) ;
#12197=CARTESIAN_POINT ( 'NONE',  ( 103.0997794884429197, 5.417593104495392886, -5.187149597110491506 ) ) ;
#12215=CARTESIAN_POINT ( 'NONE',  ( 100.1711952389851348, -3.105058450138034498, -6.829076936735990699 ) ) ;
#12231=DIRECTION ( 'NONE',  ( -0.000000000000000000, -0.000000000000000000, 1.000000000000000000 ) ) ;
#12265=EDGE_LOOP ( 'NONE', ( #18382, #900, #21636, #4815, #7043, #20019, #16103, #251, #11049, #26645, #22308, #8853 ) ) ;
#12280=CARTESIAN_POINT ( 'NONE',  ( 110.7380848894536598, 7.027127293105233764E-16, 12.50000000000000000 ) ) ;
#12283=DIRECTION ( 'NONE',  ( 0.000000000000000000, 0.000000000000000000, 1.000000000000000000 ) ) ;
#12289=CARTESIAN_POINT ( 'NONE',  ( 212.5000000000000000, 0.000000000000000000, 0.000000000000000000 ) ) ;
#12310=ORIENTED_EDGE ( 'NONE', *, *, #25748, .F. ) ;
#12316=VERTEX_POINT ( 'NONE', #5530 ) ;
#12354=DIRECTION ( 'NONE',  ( -0.000000000000000000, 0.000000000000000000, -1.000000000000000000 ) ) ;
#12364=CARTESIAN_POINT ( 'NONE',  ( 129.3530333899765594, -6.000000000000000000, -62.49999999999999289 ) ) ;
#12385=CARTESIAN_POINT ( 'NONE',  ( 108.7736657769335409, -4.337494364694277849, -6.125882734748267389 ) ) ;
#12430=CARTESIAN_POINT ( 'NONE',  ( 109.5537947374686496, -3.510783659749455499, 12.00105596243589545 ) ) ;
#12455=DIRECTION ( 'NONE',  ( -0.000000000000000000, -0.000000000000000000, 1.000000000000000000 ) ) ;
#12457=CARTESIAN_POINT ( 'NONE',  ( -110.1150203881707625, 0.3420146137956290300, -12.50000000000000000 ) ) ;
#12461=DIRECTION ( 'NONE',  ( -1.000000000000000000, 0.000000000000000000, 0.000000000000000000 ) ) ;
#12513=ORIENTED_EDGE ( 'NONE', *, *, #8543, .T. ) ;
#12548=ORIENTED_EDGE ( 'NONE', *, *, #18123, .T. ) ;
#12563=LINE ( 'NONE', #6505, #7304 ) ;
#12596=CARTESIAN_POINT ( 'NONE',  ( 99.86168570827183544, -2.560920621327513746, 12.23601723495363380 ) ) ;
#12620=EDGE_LOOP ( 'NONE', ( #29355, #18631, #22360, #6765 ) ) ;
#12640=ADVANCED_FACE ( 'NONE', ( #7775 ), #11630, .F. ) ;
#12643=B_SPLINE_CURVE_WITH_KNOTS ( 'NONE', 3,
 ( #12280, #30953, #14422, #23130, #9758, #6380, #4050, #17978, #6731, #28628, #1229, #28104, #14601, #22944, #25246, #33972, #22769, #28287, #9595, #3881, #4230, #14774, #12102, #11748, #9426, #20281, #31133, #17625, #28454, #14945, #20452, #31294, #17796, #25961, #34317, #4568, #29152, #31989, #2441, #10110, #4748, #23814 ),
 .UNSPECIFIED., .F., .F.,
 ( 4, 2, 2, 2, 2, 2, 2, 2, 2, 2, 2, 2, 2, 2, 2, 2, 2, 2, 2, 2, 4 ),
 ( 6.816353745294061091E-19, 0.001137415812192694954, 0.002274831624385389474, 0.003412247436578083343, 0.003980955342674430061, 0.004549663248770777213, 0.005687079060963441159, 0.006824494873156104237, 0.007393202779252454858, 0.007961910685348804612, 0.009099326497541465955, 0.009668034403637816576, 0.01023674230973416720, 0.01137415812192686844, 0.01251157393411956795, 0.01364898974631226745, 0.01478640555850496870, 0.01535511346460131932, 0.01592382137069766820, 0.01706123718289036598, 0.01819865299508306375 ),
 .UNSPECIFIED. ) ;
#12645=CARTESIAN_POINT ( 'NONE',  ( 212.5000000000000000, 9.184850993605147944E-16, -7.500000000000000000 ) ) ;
#12646=CARTESIAN_POINT ( 'NONE',  ( 109.5190789905360447, -3.554721378204152682, 6.612463615769124559 ) ) ;
#12651=CARTESIAN_POINT ( 'NONE',  ( 129.3530333899765594, -6.000000000000000000, -62.49999999999999289 ) ) ;
#12671=AXIS2_PLACEMENT_3D ( 'NONE', #1411, #17799, #12283 ) ;
#12685=ORIENTED_EDGE ( 'NONE', *, *, #25748, .T. ) ;
#12717=CARTESIAN_POINT ( 'NONE',  ( -105.1752859088571626, 5.114965439436506500, -5.485173521317547873 ) ) ;
#12721=CARTESIAN_POINT ( 'NONE',  ( 109.8671414378377165, 3.044914778013033452, -12.12453154756074092 ) ) ;
#12777=CARTESIAN_POINT ( 'NONE',  ( 109.8638085254334982, -3.050121699374164219, 12.12320065612944475 ) ) ;
#12782=CARTESIAN_POINT ( 'NONE',  ( -100.9573452668279003, -3.150844840328200558, -6.812360382669040426 ) ) ;
#12862=CARTESIAN_POINT ( 'NONE',  ( 117.4999999999998579, 0.000000000000000000, 0.000000000000000000 ) ) ;
#12866=ORIENTED_EDGE ( 'NONE', *, *, #6057, .F. ) ;
#12891=CARTESIAN_POINT ( 'NONE',  ( 106.9022939876274592, 5.416883352271473662, -5.187895480218550404 ) ) ;
#12893=CARTESIAN_POINT ( 'NONE',  ( -104.3114314540143965, 5.080227507390846498, -5.518150456212834953 ) ) ;
#12898=CARTESIAN_POINT ( 'NONE',  ( 100.6912675671779880, 3.794064876973125777, -11.91123467351735776 ) ) ;
#12951=CARTESIAN_POINT ( 'NONE',  ( 103.4895502457613645, -5.548707632555107239, 11.20129239819138789 ) ) ;
#12956=CARTESIAN_POINT ( 'NONE',  ( -99.92868254684908891, -0.6892679340434103574, -7.470251853870532699 ) ) ;
#12977=AXIS2_PLACEMENT_3D ( 'NONE', #29041, #4301, #26375 ) ;
#12981=DIRECTION ( 'NONE',  ( 0.000000000000000000, 0.000000000000000000, -1.000000000000000000 ) ) ;
#13014=AXIS2_PLACEMENT_3D ( 'NONE', #20603, #31115, #12083 ) ;
#13044=DIRECTION ( 'NONE',  ( -1.000000000000000000, 0.000000000000000000, 0.000000000000000000 ) ) ;
#13056=AXIS2_PLACEMENT_3D ( 'NONE', #29235, #23718, #34576 ) ;
#13073=DIRECTION ( 'NONE',  ( 1.000000000000000000, 0.000000000000000000, 0.000000000000000000 ) ) ;
#13102=DIRECTION ( 'NONE',  ( 0.000000000000000000, -1.000000000000000000, 0.000000000000000000 ) ) ;
#13122=CARTESIAN_POINT ( 'NONE',  ( -106.6942439354515955, -4.837552664684794834, -5.733718144795174609 ) ) ;
#13148=FACE_OUTER_BOUND ( 'NONE', #7583, .T. ) ;
#13162=ORIENTED_EDGE ( 'NONE', *, *, #31469, .T. ) ;
#13200=ADVANCED_FACE ( 'NONE', ( #14509 ), #24978, .T. ) ;
#13236=CARTESIAN_POINT ( 'NONE',  ( -262.5000000000000000, 1.224646799147353256E-15, -10.00000000000000000 ) ) ;
#13243=CARTESIAN_POINT ( 'NONE',  ( 99.30025296260937751, 0.7624844131070424025, -12.48227001241056655 ) ) ;
#13266=PLANE ( 'NONE',  #3931 ) ;
#13267=FACE_OUTER_BOUND ( 'NONE', #20170, .T. ) ;
#13297=CARTESIAN_POINT ( 'NONE',  ( -106.3655922539543326, 4.941456866685308924, 5.642756420309243737 ) ) ;
#13299=FACE_BOUND ( 'NONE', #33843, .T. ) ;
#13305=CARTESIAN_POINT ( 'NONE',  ( -107.5877143847361452, -4.424201595130941023, -6.060139114164995178 ) ) ;
#13325=AXIS2_PLACEMENT_3D ( 'NONE', #32318, #18646, #34654 ) ;
#13329=CARTESIAN_POINT ( 'NONE',  ( -108.1248180926981632, 4.063332493481114582, -11.82279441766105599 ) ) ;
#13350=CARTESIAN_POINT ( 'NONE',  ( -102.6980701398429403, -4.579683091146231178, 5.941712070794215705 ) ) ;
#13351=VERTEX_POINT ( 'NONE', #25757 ) ;
#13377=ORIENTED_EDGE ( 'NONE', *, *, #31577, .T. ) ;
#13403=ORIENTED_EDGE ( 'NONE', *, *, #8543, .F. ) ;
#13408=DIRECTION ( 'NONE',  ( -1.000000000000000000, 0.000000000000000000, 0.000000000000000000 ) ) ;
#13426=ORIENTED_EDGE ( 'NONE', *, *, #3698, .F. ) ;
#13427=ORIENTED_EDGE ( 'NONE', *, *, #31469, .F. ) ;
#13464=CARTESIAN_POINT ( 'NONE',  ( -107.2958507442938014, 4.573766672917669140, 5.944761500833684487 ) ) ;
#13466=ORIENTED_EDGE ( 'NONE', *, *, #25680, .T. ) ;
#13469=CARTESIAN_POINT ( 'NONE',  ( -100.6805073636512589, -2.744499711777490081, -6.981349484866706590 ) ) ;
#13494=CARTESIAN_POINT ( 'NONE',  ( -100.5730760456114865, 2.567831768330361530, -12.23432884111322316 ) ) ;
#13497=AXIS2_PLACEMENT_3D ( 'NONE', #31591, #25909, #10059 ) ;
#13501=LINE ( 'NONE', #24336, #3148 ) ;
#13524=CARTESIAN_POINT ( 'NONE',  ( 99.26191511054601335, -2.804307960831458189E-14, 7.500000000000241585 ) ) ;
#13528=VERTEX_POINT ( 'NONE', #18131 ) ;
#13543=AXIS2_PLACEMENT_3D ( 'NONE', #907, #27947, #19427 ) ;
#13544=EDGE_CURVE ( 'NONE', #30505, #9756, #33108, .T. ) ;
#13609=CARTESIAN_POINT ( 'NONE',  ( 109.6573908833661903, -3.356891575080633849, -12.04186941445821724 ) ) ;
#13618=EDGE_CURVE ( 'NONE', #8598, #5515, #26987, .T. ) ;
#13625=ORIENTED_EDGE ( 'NONE', *, *, #23297, .T. ) ;
#13626=EDGE_CURVE ( 'NONE', #17170, #549, #843, .T. ) ;
#13632=FACE_OUTER_BOUND ( 'NONE', #13646, .T. ) ;
#13646=EDGE_LOOP ( 'NONE', ( #22529, #195, #3986, #25537 ) ) ;
#13647=DIRECTION ( 'NONE',  ( -1.000000000000000000, -0.000000000000000000, -0.000000000000000000 ) ) ;
#13662=CARTESIAN_POINT ( 'NONE',  ( -109.9487023029381589, 1.336696757081942799, -12.43272095415539624 ) ) ;
#13680=EDGE_CURVE ( 'NONE', #14310, #3870, #22729, .T. ) ;
#13683=CARTESIAN_POINT ( 'NONE',  ( -105.3468572192119694, -5.115148824049938092, 5.485002510375799112 ) ) ;
#13724=CARTESIAN_POINT ( 'NONE',  ( 106.3567858119077840, 5.578687132273540961, 5.013157219915588492 ) ) ;
#13741=PLANE ( 'NONE',  #9939 ) ;
#13749=ADVANCED_FACE ( 'NONE', ( #22175 ), #4117, .T. ) ;
#13793=ORIENTED_EDGE ( 'NONE', *, *, #2471, .F. ) ;
#13822=CARTESIAN_POINT ( 'NONE',  ( -119.9999999999997726, 1.224646799147353256E-15, -10.00000000000000000 ) ) ;
#13826=LINE ( 'NONE', #826, #4271 ) ;
#13845=CARTESIAN_POINT ( 'NONE',  ( -100.9384238677276358, 3.126956236148901169, -12.10589691785417976 ) ) ;
#13863=CARTESIAN_POINT ( 'NONE',  ( -109.8381179908438554, -1.694081942180569733, 7.313267332261218279 ) ) ;
#13875=EDGE_CURVE ( 'NONE', #19820, #30104, #5112, .T. ) ;
#13878=ORIENTED_EDGE ( 'NONE', *, *, #435, .T. ) ;
#13905=CARTESIAN_POINT ( 'NONE',  ( 105.3927003681590548, 5.728044018051756225, 4.841538128164400767 ) ) ;
#13916=EDGE_CURVE ( 'NONE', #12316, #3925, #2529, .T. ) ;
#14042=CARTESIAN_POINT ( 'NONE',  ( -100.8614468863726756, -3.010446655309094499, 6.870869395578496963 ) ) ;
#14061=ORIENTED_EDGE ( 'NONE', *, *, #31180, .F. ) ;
#14143=CARTESIAN_POINT ( 'NONE',  ( 110.5494250287361808, -1.507735446164279125, -12.41434713890700969 ) ) ;
#14158=FACE_OUTER_BOUND ( 'NONE', #4034, .T. ) ;
#14185=EDGE_LOOP ( 'NONE', ( #4311, #21070, #8093, #3665 ) ) ;
#14193=EDGE_CURVE ( 'NONE', #11373, #8598, #23837, .T. ) ;
#14194=EDGE_CURVE ( 'NONE', #3925, #12316, #2896, .T. ) ;
#14200=EDGE_CURVE ( 'NONE', #549, #17170, #9285, .T. ) ;
#14244=AXIS2_PLACEMENT_3D ( 'NONE', #12862, #28863, #21206 ) ;
#14247=CARTESIAN_POINT ( 'NONE',  ( 129.3530333899765594, -6.000000000000000000, 57.49999999999999289 ) ) ;
#14263=CARTESIAN_POINT ( 'NONE',  ( 102.4121716945766565, 5.134660333356495521, 5.470525374126623319 ) ) ;
#14268=CARTESIAN_POINT ( 'NONE',  ( -99.88497961182919482, 6.264410040187948829E-16, -12.50000000000000000 ) ) ;
#14290=LINE ( 'NONE', #21751, #3260 ) ;
#14304=CIRCLE ( 'NONE', #33618, 5.115020388170798959 ) ;
#14308=VERTEX_POINT ( 'NONE', #11909 ) ;
#14309=LINE ( 'NONE', #12645, #25817 ) ;
#14310=VERTEX_POINT ( 'NONE', #33597 ) ;
#14325=CARTESIAN_POINT ( 'NONE',  ( 108.7902275512028751, -4.324042002361276005, -11.73155476838175204 ) ) ;
#14328=ORIENTED_EDGE ( 'NONE', *, *, #2430, .F. ) ;
#14341=CARTESIAN_POINT ( 'NONE',  ( 103.4594491513664849, 5.530628908288163004, -5.066456342206738128 ) ) ;
#14390=CARTESIAN_POINT ( 'NONE',  ( -100.1515056346334944, 1.663653002832651495, 12.39274845084345422 ) ) ;
#14399=ADVANCED_FACE ( 'NONE', ( #32155 ), #4553, .T. ) ;
#14417=VERTEX_POINT ( 'NONE', #7581 ) ;
#14422=CARTESIAN_POINT ( 'NONE',  ( 110.6997470373906225, 0.7624844131070430686, 12.48227001241056833 ) ) ;
#14435=CARTESIAN_POINT ( 'NONE',  ( -101.8747319636630522, -4.062792622693891076, 11.82295934283893324 ) ) ;
#14509=FACE_OUTER_BOUND ( 'NONE', #30095, .T. ) ;
#14561=VERTEX_POINT ( 'NONE', #10802 ) ;
#14601=CARTESIAN_POINT ( 'NONE',  ( 108.5051184359966214, 4.558408617645862471, 11.64136836827557886 ) ) ;
#14619=ORIENTED_EDGE ( 'NONE', *, *, #15807, .F. ) ;
#14695=CARTESIAN_POINT ( 'NONE',  ( 99.88047028666090910, 2.618976401886136340, -7.037310091161540271 ) ) ;
#14708=AXIS2_PLACEMENT_3D ( 'NONE', #28092, #11557, #8692 ) ;
#14713=CARTESIAN_POINT ( 'NONE',  ( 106.9079130804741595, -5.424061631995436450, -5.183681401394261812 ) ) ;
#14742=CARTESIAN_POINT ( 'NONE',  ( -103.3401862807116629, 4.841160850826510043, 11.52458411820204276 ) ) ;
#14774=CARTESIAN_POINT ( 'NONE',  ( 104.8142247405124152, 5.738231822805250459, 11.10507521702373879 ) ) ;
#14794=FACE_BOUND ( 'NONE', #27925, .T. ) ;
#14800=CARTESIAN_POINT ( 'NONE',  ( -109.0561609099978142, -3.120668149329707042, -12.10491939767606873 ) ) ;
#14815=LINE ( 'NONE', #9287, #8374 ) ;
#14831=EDGE_CURVE ( 'NONE', #17516, #731, #26073, .T. ) ;
#14838=ORIENTED_EDGE ( 'NONE', *, *, #20666, .F. ) ;
#14853=DIRECTION ( 'NONE',  ( -1.000000000000000000, 0.000000000000000000, 0.000000000000000000 ) ) ;
#14864=CARTESIAN_POINT ( 'NONE',  ( 100.7130364623890131, 3.831042253767035444, -6.454752727393734624 ) ) ;
#14882=CARTESIAN_POINT ( 'NONE',  ( 105.7869846758901815, -5.687305096039679597, -4.889329717555864541 ) ) ;
#14892=ORIENTED_EDGE ( 'NONE', *, *, #7487, .F. ) ;
#14945=CARTESIAN_POINT ( 'NONE',  ( 101.4934480377529979, 4.557154561855115027, 11.64184170122662287 ) ) ;
#14958=ORIENTED_EDGE ( 'NONE', *, *, #3698, .T. ) ;
#15006=DIRECTION ( 'NONE',  ( -0.000000000000000000, -0.000000000000000000, -1.000000000000000000 ) ) ;
#15039=CARTESIAN_POINT ( 'NONE',  ( -105.8665330455879143, 5.043966910541457516, -5.550724164612919509 ) ) ;
#15055=CARTESIAN_POINT ( 'NONE',  ( 103.4525503535520414, -5.538930788889586232, -5.058095442343715220 ) ) ;
#15079=ORIENTED_EDGE ( 'NONE', *, *, #15807, .T. ) ;
#15087=CARTESIAN_POINT ( 'NONE',  ( -109.9476871814112684, 1.341502966352549508, 12.43231302123709625 ) ) ;
#15095=CARTESIAN_POINT ( 'NONE',  ( 100.8159517847998075, -3.931125184197652445, 11.86656790805995243 ) ) ;
#15130=DIRECTION ( 'NONE',  ( -0.000000000000000000, 1.000000000000000000, -0.000000000000000000 ) ) ;
#15195=FACE_OUTER_BOUND ( 'NONE', #12620, .T. ) ;
#15209=CARTESIAN_POINT ( 'NONE',  ( -102.8541734989807424, 4.646131333787439921, -5.888157618374222579 ) ) ;
#15216=CARTESIAN_POINT ( 'NONE',  ( 101.4948815640033928, 4.558408617645864247, -11.64136836827557708 ) ) ;
#15261=CARTESIAN_POINT ( 'NONE',  ( -109.3398582488967890, 2.712336548677834802, 12.20300697856196059 ) ) ;
#15271=CARTESIAN_POINT ( 'NONE',  ( 102.1097078945684444, -4.970825052104117070, 11.47130252761374614 ) ) ;
#15275=CARTESIAN_POINT ( 'NONE',  ( 129.3530333899765594, -6.000000000000000000, 57.49999999999999289 ) ) ;
#15318=CARTESIAN_POINT ( 'NONE',  ( 99.26191511054629757, -0.1972643383979439669, 7.500000000000013323 ) ) ;
#15323=CARTESIAN_POINT ( 'NONE',  ( -110.1150203881707910, 3.166944581793445397E-20, 12.50000000000000000 ) ) ;
#15369=ADVANCED_FACE ( 'NONE', ( #696 ), #30067, .T. ) ;
#15372=DIRECTION ( 'NONE',  ( 0.000000000000000000, 0.000000000000000000, 1.000000000000000000 ) ) ;
#15381=CARTESIAN_POINT ( 'NONE',  ( 106.3573986772276498, 5.578557642680240569, -5.013303406467239931 ) ) ;
#15406=ADVANCED_FACE ( 'NONE', ( #5834 ), #20553, .T. ) ;
#15442=CARTESIAN_POINT ( 'NONE',  ( 107.8890288426244410, -4.971563738489883200, 11.47098163371368251 ) ) ;
#15471=DIRECTION ( 'NONE',  ( -0.000000000000000000, -0.000000000000000000, -1.000000000000000000 ) ) ;
#15473=ORIENTED_EDGE ( 'NONE', *, *, #29645, .T. ) ;
#15490=CARTESIAN_POINT ( 'NONE',  ( 101.5068632955307208, -4.566352457759228045, 5.955250171528614800 ) ) ;
#15507=DIRECTION ( 'NONE',  ( -0.7071067811865435759, 0.000000000000000000, 0.7071067811865514585 ) ) ;
#15522=ORIENTED_EDGE ( 'NONE', *, *, #33879, .F. ) ;
#15540=FACE_OUTER_BOUND ( 'NONE', #20450, .T. ) ;
#15542=FACE_OUTER_BOUND ( 'NONE', #16534, .T. ) ;
#15546=ORIENTED_EDGE ( 'NONE', *, *, #25588, .F. ) ;
#15553=CARTESIAN_POINT ( 'NONE',  ( -107.3021478268368014, 4.579603235088350210, -5.941779048586183443 ) ) ;
#15559=CARTESIAN_POINT ( 'NONE',  ( 105.9472385653803173, 5.662516510817760640, -11.14395138485681436 ) ) ;
#15618=CARTESIAN_POINT ( 'NONE',  ( 212.5000000000000000, 1.224646799147353256E-15, -10.00000000000000000 ) ) ;
#15623=CARTESIAN_POINT ( 'NONE',  ( 99.56119438876471861, -1.867505626284030162, 12.36477516193776260 ) ) ;
#15627=CARTESIAN_POINT ( 'NONE',  ( -101.8763945071601285, -4.063426306576022995, -6.307665442424296387 ) ) ;
#15656=ADVANCED_FACE ( 'NONE', ( #9928 ), #18489, .F. ) ;
#15659=LINE ( 'NONE', #33982, #8813 ) ;
#15671=CARTESIAN_POINT ( 'NONE',  ( 105.3950378164618229, -5.727834534852265236, 4.841784820303065118 ) ) ;
#15672=CIRCLE ( 'NONE', #4840, 10.00000000000000000 ) ;
#15684=EDGE_LOOP ( 'NONE', ( #6362, #28839, #32832, #26997 ) ) ;
#15712=ORIENTED_EDGE ( 'NONE', *, *, #4030, .T. ) ;
#15802=CARTESIAN_POINT ( 'NONE',  ( 110.5486025016846412, -1.510413401456684790, 12.41397948795683526 ) ) ;
#15804=CARTESIAN_POINT ( 'NONE',  ( 212.5000000000000000, 0.000000000000000000, 0.000000000000000000 ) ) ;
#15807=EDGE_CURVE ( 'NONE', #30104, #19820, #16607, .T. ) ;
#15809=CARTESIAN_POINT ( 'NONE',  ( -99.89370470387717660, -0.3451077285824861729, -7.494041212912380345 ) ) ;
#15832=CARTESIAN_POINT ( 'NONE',  ( -105.3411554791202036, 5.114806216612618250, -11.40564585725304170 ) ) ;
#15836=FACE_OUTER_BOUND ( 'NONE', #11940, .T. ) ;
#15851=CARTESIAN_POINT ( 'NONE',  ( 100.7152960566303364, -3.833500081834649187, 6.453260708061876905 ) ) ;
#15890=LINE ( 'NONE', #2323, #3482 ) ;
#15895=CARTESIAN_POINT ( 'NONE',  ( 110.7380848894536598, 0.3991779689724688773, 7.500000000000000000 ) ) ;
#15909=CYLINDRICAL_SURFACE ( 'NONE', #13056, 5.115020388170798959 ) ;
#15917=LINE ( 'NONE', #10561, #16813 ) ;
#15966=CARTESIAN_POINT ( 'NONE',  ( -110.1150203881707910, 0.000000000000000000, 57.49999999999999289 ) ) ;
#15972=CARTESIAN_POINT ( 'NONE',  ( -100.1627706953726005, 1.696271239234545813, 7.312686146626633743 ) ) ;
#15976=CARTESIAN_POINT ( 'NONE',  ( -100.0598114771552929, -1.370240552585038962, -7.381692049079064510 ) ) ;
#15998=CARTESIAN_POINT ( 'NONE',  ( -99.88497961182919482, 6.264410040187948829E-16, -12.50000000000000000 ) ) ;
#16019=DIRECTION ( 'NONE',  ( -1.000000000000000000, 0.000000000000000000, 0.000000000000000000 ) ) ;
#16020=CARTESIAN_POINT ( 'NONE',  ( 99.88220250681632706, -2.622468385745837072, 7.036045090041716854 ) ) ;
#16053=ORIENTED_EDGE ( 'NONE', *, *, #25264, .F. ) ;
#16103=ORIENTED_EDGE ( 'NONE', *, *, #27361, .T. ) ;
#16109=CYLINDRICAL_SURFACE ( 'NONE', #30014, 5.115020388170798959 ) ;
#16148=LINE ( 'NONE', #15618, #30943 ) ;
#16151=CARTESIAN_POINT ( 'NONE',  ( -109.1385531136273670, -3.010446655309096720, -6.870869395578498739 ) ) ;
#16197=CARTESIAN_POINT ( 'NONE',  ( -102.4122856152638406, -4.424201595130935694, 6.060139114165001395 ) ) ;
#16203=CARTESIAN_POINT ( 'NONE',  ( -107.5838244394680032, 4.417479313406522223, 6.061799023038634715 ) ) ;
#16207=CARTESIAN_POINT ( 'NONE',  ( -99.88497961182919482, 6.264093345946822590E-16, -57.49999999999999289 ) ) ;
#16211=AXIS2_PLACEMENT_3D ( 'NONE', #5155, #32748, #27411 ) ;
#16267=DIRECTION ( 'NONE',  ( -0.000000000000000000, -0.000000000000000000, -1.000000000000000000 ) ) ;
#16269=EDGE_LOOP ( 'NONE', ( #22716, #22583, #14892, #5252 ) ) ;
#16285=DIRECTION ( 'NONE',  ( -1.000000000000000000, 0.000000000000000000, 0.000000000000000000 ) ) ;
#16294=CARTESIAN_POINT ( 'NONE',  ( 99.30126570083648119, -0.7699128213881771821, -12.48180554319666236 ) ) ;
#16326=CARTESIAN_POINT ( 'NONE',  ( -109.9396462212316266, 1.371756618311864795, 7.381329779211299957 ) ) ;
#16337=VECTOR ( 'NONE', #8474, 1000.000000000000000 ) ;
#16345=CARTESIAN_POINT ( 'NONE',  ( 129.3530333899765594, 6.000000000000000000, -62.49999999999999289 ) ) ;
#16357=CARTESIAN_POINT ( 'NONE',  ( -106.1720655868554530, 4.981785521925212734, -11.46442881298733063 ) ) ;
#16360=VERTEX_POINT ( 'NONE', #3092 ) ;
#16366=ADVANCED_FACE ( 'NONE', ( #13267 ), #7911, .T. ) ;
#16388=EDGE_LOOP ( 'NONE', ( #2270, #14328, #33048, #9732 ) ) ;
#16400=CARTESIAN_POINT ( 'NONE',  ( 129.3530333899765594, 6.000000000000000000, -62.49999999999999289 ) ) ;
#16411=ADVANCED_FACE ( 'NONE', ( #3793, #23030 ), #28191, .T. ) ;
#16418=CARTESIAN_POINT ( 'NONE',  ( 103.0977060123724698, 5.416883352271473662, 5.187895480218550404 ) ) ;
#16429=FACE_OUTER_BOUND ( 'NONE', #16269, .T. ) ;
#16447=CARTESIAN_POINT ( 'NONE',  ( 110.6869025488327196, -0.7897130297925551989, -7.460902677354920520 ) ) ;
#16451=ORIENTED_EDGE ( 'NONE', *, *, #18858, .F. ) ;
#16469=CARTESIAN_POINT ( 'NONE',  ( 109.3101759974547633, -3.792433597769626630, -11.91175651985687622 ) ) ;
#16495=ORIENTED_EDGE ( 'NONE', *, *, #2037, .F. ) ;
#16504=ADVANCED_FACE ( 'NONE', ( #20012, #6459, #15542 ), #20525, .F. ) ;
#16528=CARTESIAN_POINT ( 'NONE',  ( -100.3431920928583736, 2.122570655097208547, -12.31945284403700569 ) ) ;
#16534=EDGE_LOOP ( 'NONE', ( #5329, #4237, #11301, #11573 ) ) ;
#16589=CARTESIAN_POINT ( 'NONE',  ( 99.88736582462350100, 2.611822472857947108, 7.032742872185955285 ) ) ;
#16607=CIRCLE ( 'NONE', #2290, 12.50000000000000000 ) ;
#16610=FACE_OUTER_BOUND ( 'NONE', #26643, .T. ) ;
#16619=CARTESIAN_POINT ( 'NONE',  ( -101.6271750261120417, 3.859208454723694892, -6.436243333213718998 ) ) ;
#16628=( LENGTH_UNIT ( ) NAMED_UNIT ( * ) SI_UNIT ( .MILLI., .METRE. ) );
#16646=CARTESIAN_POINT ( 'NONE',  ( 103.4959836398287649, -5.550599894338584583, -11.20035359757824089 ) ) ;
#16651=ADVANCED_FACE ( 'NONE', ( #15195 ), #20704, .T. ) ;
#16671=VERTEX_POINT ( 'NONE', #1823 ) ;
#16705=CARTESIAN_POINT ( 'NONE',  ( -106.6587923562685916, 4.850327849261239166, 11.52145900171629656 ) ) ;
#16723=CARTESIAN_POINT ( 'NONE',  ( -100.9608953138632899, -3.142556659824618404, 6.811296903636076649 ) ) ;
#16748=CARTESIAN_POINT ( 'NONE',  ( -119.9999999999997726, 0.000000000000000000, 10.00000000000000000 ) ) ;
#16768=CARTESIAN_POINT ( 'NONE',  ( 105.7860010550761416, 5.687433884741868617, 4.889179432777876144 ) ) ;
#16781=CARTESIAN_POINT ( 'NONE',  ( 117.4999999999998579, 0.000000000000000000, 12.50000000000000000 ) ) ;
#16813=VECTOR ( 'NONE', #29593, 1000.000000000000000 ) ;
#16834=ORIENTED_EDGE ( 'NONE', *, *, #14194, .F. ) ;
#16878=CONICAL_SURFACE ( 'NONE', #8336, 12.50000000000000000, 0.7853981633974431720 ) ;
#16883=CARTESIAN_POINT ( 'NONE',  ( -262.5000000000000000, 9.184850993605147944E-16, -7.500000000000000000 ) ) ;
#16932=CARTESIAN_POINT ( 'NONE',  ( -102.4259574044266543, -4.432593925698492754, 11.68934397677213965 ) ) ;
#16949=CARTESIAN_POINT ( 'NONE',  ( 100.7111166766537735, 3.828784459365716319, 6.456053091683092049 ) ) ;
#16958=ORIENTED_EDGE ( 'NONE', *, *, #10853, .F. ) ;
#16962=DIRECTION ( 'NONE',  ( 1.000000000000000000, 0.000000000000000000, 0.000000000000000000 ) ) ;
#17004=CARTESIAN_POINT ( 'NONE',  ( 100.4462052625313646, -3.510783659749458607, -12.00105596243589723 ) ) ;
#17007=CARTESIAN_POINT ( 'NONE',  ( -262.5000000000000000, 0.000000000000000000, 0.000000000000000000 ) ) ;
#17009=CARTESIAN_POINT ( 'NONE',  ( 212.5000000000000000, 0.000000000000000000, 10.00000000000000000 ) ) ;
#17018=CARTESIAN_POINT ( 'NONE',  ( 99.58104344416952358, 1.924456215511286983, -7.258046499395033102 ) ) ;
#17097=LINE ( 'NONE', #27930, #31404 ) ;
#17101=CARTESIAN_POINT ( 'NONE',  ( 127.4999999999999147, 3.061616997868169163E-16, -2.499999999999825473 ) ) ;
#17104=CARTESIAN_POINT ( 'NONE',  ( -109.8494042611863506, -1.661087400543260317, 12.39310421627767766 ) ) ;
#17115=PLANE ( 'NONE',  #13543 ) ;
#17170=VERTEX_POINT ( 'NONE', #28084 ) ;
#17189=DIRECTION ( 'NONE',  ( -1.000000000000000000, 0.000000000000000000, 0.000000000000000000 ) ) ;
#17277=ORIENTED_EDGE ( 'NONE', *, *, #24304, .T. ) ;
#17286=VECTOR ( 'NONE', #30964, 1000.000000000000000 ) ;
#17287=CARTESIAN_POINT ( 'NONE',  ( -100.8451065690243951, -2.987912174852660474, 12.13846169321888979 ) ) ;
#17295=ORIENTED_EDGE ( 'NONE', *, *, #19368, .F. ) ;
#17318=DIRECTION ( 'NONE',  ( -1.000000000000000000, 0.000000000000000000, 0.000000000000000000 ) ) ;
#17326=AXIS2_PLACEMENT_3D ( 'NONE', #15804, #26636, #10628 ) ;
#17330=DIRECTION ( 'NONE',  ( 0.000000000000000000, -1.000000000000000000, 0.000000000000000000 ) ) ;
#17336=( NAMED_UNIT ( * ) PLANE_ANGLE_UNIT ( ) SI_UNIT ( $, .RADIAN. ) );
#17373=CARTESIAN_POINT ( 'NONE',  ( 104.0198594782632853, 5.657025933901884684, -4.924586583110066584 ) ) ;
#17390=CARTESIAN_POINT ( 'NONE',  ( 104.8009589134950232, -5.738006884272855324, -4.829624934769205069 ) ) ;
#17402=ADVANCED_FACE ( 'NONE', ( #23795, #13299, #18816 ), #10970, .F. ) ;
#17414=CARTESIAN_POINT ( 'NONE',  ( -99.88497961182919482, 6.264093345946821604E-16, 12.50000000000000000 ) ) ;
#17417=LINE ( 'NONE', #22735, #26300 ) ;
#17469=EDGE_CURVE ( 'NONE', #2593, #25686, #16148, .T. ) ;
#17470=CARTESIAN_POINT ( 'NONE',  ( -99.88497961182919482, 6.264093345946821604E-16, 12.50000000000000000 ) ) ;
#17479=EDGE_CURVE ( 'NONE', #16, #21237, #33765, .T. ) ;
#17487=CARTESIAN_POINT ( 'NONE',  ( -105.3361376941048064, -5.115085776248457172, -11.40552048381710115 ) ) ;
#17508=AXIS2_PLACEMENT_3D ( 'NONE', #10905, #24772, #11086 ) ;
#17516=VERTEX_POINT ( 'NONE', #30356 ) ;
#17592=CARTESIAN_POINT ( 'NONE',  ( -109.5852389964325369, 2.273103392716669724, 12.29250028061669120 ) ) ;
#17599=DIRECTION ( 'NONE',  ( -0.000000000000000000, -0.000000000000000000, 1.000000000000000000 ) ) ;
#17625=CARTESIAN_POINT ( 'NONE',  ( 102.4375534982951592, 5.148005685260262254, 11.39183432441182653 ) ) ;
#17652=AXIS2_PLACEMENT_3D ( 'NONE', #9819, #33008, #5956 ) ;
#17727=CARTESIAN_POINT ( 'NONE',  ( 100.0742843969711231, -2.949151772667967020, -6.898053038626237310 ) ) ;
#17743=CIRCLE ( 'NONE', #9736, 5.738084889453667792 ) ;
#17769=CARTESIAN_POINT ( 'NONE',  ( 100.1355683589712271, -3.049149995829645743, 12.12344935835687387 ) ) ;
#17796=CARTESIAN_POINT ( 'NONE',  ( 100.4456562794407404, 3.510468032099187230, 12.00123740321143728 ) ) ;
#17799=DIRECTION ( 'NONE',  ( -1.000000000000000000, -0.000000000000000000, -0.000000000000000000 ) ) ;
#17897=CARTESIAN_POINT ( 'NONE',  ( 99.85295625471279379, 2.564129753321951366, -12.23925059504672497 ) ) ;
#17916=VERTEX_POINT ( 'NONE', #7890 ) ;
#17962=LINE ( 'NONE', #9219, #33819 ) ;
#17978=CARTESIAN_POINT ( 'NONE',  ( 109.6574619143216580, 3.356865266134899439, 12.04189187465341959 ) ) ;
#17987=CARTESIAN_POINT ( 'NONE',  ( -262.5000000000000000, 0.000000000000000000, 0.000000000000000000 ) ) ;
#17994=ORIENTED_EDGE ( 'NONE', *, *, #23931, .F. ) ;
#17995=B_SPLINE_CURVE_WITH_KNOTS ( 'NONE', 3,
 ( #4238, #12457, #137, #13662, #2447, #31994, #8139, #19199, #30040, #21332, #13329, #2797, #29341, #32702, #24160, #21669, #16357, #7605, #15832, #35040, #10653, #5110, #18676, #18507, #24496, #19024, #21841, #7963, #13845, #21505, #13494, #5631, #16528, #5466, #24680, #26839, #32347, #15998 ),
 .UNSPECIFIED., .F., .F.,
 ( 4, 2, 2, 2, 2, 2, 2, 2, 2, 2, 2, 2, 2, 2, 2, 2, 2, 2, 4 ),
 ( 6.964173773746940579E-19, 0.001010717872208370584, 0.002021435744416740302, 0.003032153616625109585, 0.004042871488833478869, 0.005053589361041847285, 0.006064307233250216568, 0.006569666169354382128, 0.007075025105458547688, 0.008085742977666834572, 0.009096460849875124058, 0.01010717872208341354, 0.01111789659429170130, 0.01212861446649999078, 0.01313933233870828200, 0.01364469127481241460, 0.01415005021091654720, 0.01516076808312482802, 0.01617148595533311056 ),
 .UNSPECIFIED. ) ;
#18016=DIRECTION ( 'NONE',  ( -1.000000000000000000, 0.000000000000000000, 0.000000000000000000 ) ) ;
#18027=CARTESIAN_POINT ( 'NONE',  ( 110.7380848894536598, 7.027127293105233764E-16, 60.00000000000000000 ) ) ;
#18066=CARTESIAN_POINT ( 'NONE',  ( 107.9034705589754140, 4.962255517573300523, -5.629655879752474057 ) ) ;
#18069=CARTESIAN_POINT ( 'NONE',  ( 129.3530333899765594, -6.000000000000000000, 62.49999999999999289 ) ) ;
#18072=CARTESIAN_POINT ( 'NONE',  ( 103.4959697225922923, 5.540701522433005621, -11.20510851329257918 ) ) ;
#18099=ADVANCED_FACE ( 'NONE', ( #26022 ), #20175, .T. ) ;
#18120=CARTESIAN_POINT ( 'NONE',  ( -110.0817944407243374, 0.6742432172868401130, 12.48628981526124981 ) ) ;
#18123=EDGE_CURVE ( 'NONE', #13351, #34071, #20514, .T. ) ;
#18131=CARTESIAN_POINT ( 'NONE',  ( 99.26191511054632599, -4.118294838564020743E-16, -7.500000000000000000 ) ) ;
#18157=CARTESIAN_POINT ( 'NONE',  ( 212.5000000000000000, 0.000000000000000000, 10.00000000000000000 ) ) ;
#18161=DIRECTION ( 'NONE',  ( -1.000000000000000000, -0.000000000000000000, -0.000000000000000000 ) ) ;
#18178=PLANE ( 'NONE',  #28374 ) ;
#18189=ORIENTED_EDGE ( 'NONE', *, *, #23719, .F. ) ;
#18237=CARTESIAN_POINT ( 'NONE',  ( 110.1417579324062217, 2.553994279224888420, -12.23746534924524987 ) ) ;
#18295=CARTESIAN_POINT ( 'NONE',  ( 109.3188951714813157, -3.796349414716898796, 11.91283353888524310 ) ) ;
#18343=CARTESIAN_POINT ( 'NONE',  ( 129.3530333899765594, -6.000000000000000000, 62.49999999999999289 ) ) ;
#18382=ORIENTED_EDGE ( 'NONE', *, *, #23686, .T. ) ;
#18397=DIRECTION ( 'NONE',  ( -1.000000000000000000, 0.000000000000000000, 0.000000000000000000 ) ) ;
#18401=FACE_OUTER_BOUND ( 'NONE', #15684, .T. ) ;
#18403=CARTESIAN_POINT ( 'NONE',  ( 110.6976704948526020, 0.7843626702862538380, -7.468944954497490407 ) ) ;
#18405=CARTESIAN_POINT ( 'NONE',  ( -110.0793211855294658, 0.6938560566811355912, -7.475525031754234995 ) ) ;
#18425=ORIENTED_EDGE ( 'NONE', *, *, #14831, .T. ) ;
#18474=SHAPE_REPRESENTATION ( 'shaft', ( #28566 ), #32533 ) ;
#18476=CARTESIAN_POINT ( 'NONE',  ( 106.8634821253765637, -5.440007577125886229, 11.25529792293082032 ) ) ;
#18481=CARTESIAN_POINT ( 'NONE',  ( -106.3678849252397640, -4.940539628404770234, -5.643550520051347164 ) ) ;
#18489=CYLINDRICAL_SURFACE ( 'NONE', #29592, 7.500000000000000000 ) ;
#18500=VERTEX_POINT ( 'NONE', #29929 ) ;
#18507=CARTESIAN_POINT ( 'NONE',  ( -102.7184718528696692, 4.590414103366520671, -11.62745871345765458 ) ) ;
#18526=CYLINDRICAL_SURFACE ( 'NONE', #21880, 5.115020388170798959 ) ;
#18527=CARTESIAN_POINT ( 'NONE',  ( 106.5474496464479728, -5.538930788889586232, 5.058095442343715220 ) ) ;
#18572=DIRECTION ( 'NONE',  ( 0.000000000000000000, 0.000000000000000000, 1.000000000000000000 ) ) ;
#18592=CARTESIAN_POINT ( 'NONE',  ( 102.1149735546430435, 4.974089543361916554, -11.46991629550682035 ) ) ;
#18627=LINE ( 'NONE', #10246, #9259 ) ;
#18631=ORIENTED_EDGE ( 'NONE', *, *, #8888, .T. ) ;
#18636=VECTOR ( 'NONE', #21410, 1000.000000000000000 ) ;
#18644=CARTESIAN_POINT ( 'NONE',  ( -104.8247140911428374, 5.114965439436505612, 5.485173521317548762 ) ) ;
#18646=DIRECTION ( 'NONE',  ( 0.000000000000000000, -0.000000000000000000, 1.000000000000000000 ) ) ;
#18649=CARTESIAN_POINT ( 'NONE',  ( -108.3784044661085773, -3.854070255762958919, -6.439229133474692723 ) ) ;
#18676=CARTESIAN_POINT ( 'NONE',  ( -103.3412076437314369, 4.850327849261240054, -11.52145900171629833 ) ) ;
#18694=CARTESIAN_POINT ( 'NONE',  ( 104.2130153241097901, -5.687305096039679597, 4.889329717555864541 ) ) ;
#18724=EDGE_CURVE ( 'NONE', #6040, #32630, #119, .T. ) ;
#18725=VECTOR ( 'NONE', #12231, 1000.000000000000000 ) ;
#18760=CARTESIAN_POINT ( 'NONE',  ( 110.7380848894536598, 7.027127293105233764E-16, 60.00000000000000000 ) ) ;
#18785=CARTESIAN_POINT ( 'NONE',  ( 105.0000000000000000, 0.000000000000000000, 60.00000000000000000 ) ) ;
#18788=CARTESIAN_POINT ( 'NONE',  ( 99.26191511054632599, 0.000000000000000000, 60.00000000000000000 ) ) ;
#18814=CARTESIAN_POINT ( 'NONE',  ( -102.6978521731631702, 4.579603235088349322, 5.941779048586182554 ) ) ;
#18815=ORIENTED_EDGE ( 'NONE', *, *, #11983, .T. ) ;
#18816=FACE_OUTER_BOUND ( 'NONE', #2545, .T. ) ;
#18818=CARTESIAN_POINT ( 'NONE',  ( -105.1762619145411293, -5.114955647091113278, -5.485182652933522363 ) ) ;
#18843=VECTOR ( 'NONE', #9100, 1000.000000000000000 ) ;
#18858=EDGE_CURVE ( 'NONE', #14308, #6643, #19703, .T. ) ;
#18863=CARTESIAN_POINT ( 'NONE',  ( -107.5860917622571407, -4.424982940199791770, 6.059505149883825936 ) ) ;
#18867=EDGE_CURVE ( 'NONE', #16, #14561, #13826, .T. ) ;
#18903=CARTESIAN_POINT ( 'NONE',  ( 104.9997419262085430, 5.748131698890998287, 4.817519326574049465 ) ) ;
#18936=CARTESIAN_POINT ( 'NONE',  ( 110.4182009727613547, -1.926730348087509981, -7.257477599627513598 ) ) ;
#18958=CARTESIAN_POINT ( 'NONE',  ( 102.4443407045872902, -5.151199242560473124, -11.39037137834242586 ) ) ;
#18989=CARTESIAN_POINT ( 'NONE',  ( -108.3728249738879583, 3.859208454723701998, 6.436243333213716333 ) ) ;
#19024=CARTESIAN_POINT ( 'NONE',  ( -101.8755507196252950, 4.063381404898921190, -11.82275161328742641 ) ) ;
#19033=VECTOR ( 'NONE', #25274, 1000.000000000000000 ) ;
#19043=CARTESIAN_POINT ( 'NONE',  ( -100.2299249775011418, -1.854090048725077100, 7.268955362025008249 ) ) ;
#19061=ORIENTED_EDGE ( 'NONE', *, *, #24304, .F. ) ;
#19068=LINE ( 'NONE', #16400, #25443 ) ;
#19119=CARTESIAN_POINT ( 'NONE',  ( -130.6469666100234406, 6.000000000000000000, -62.49999999999999289 ) ) ;
#19140=CARTESIAN_POINT ( 'NONE',  ( 110.7380848894536598, -0.3789272201562005615, -12.50000000000000533 ) ) ;
#19142=VERTEX_POINT ( 'NONE', #27123 ) ;
#19169=CARTESIAN_POINT ( 'NONE',  ( -104.3031396033928218, 5.070301591678567199, 5.526538532257565528 ) ) ;
#19199=CARTESIAN_POINT ( 'NONE',  ( -109.0611100676622272, 3.127595108844668736, -12.10573782681415267 ) ) ;
#19289=CARTESIAN_POINT ( 'NONE',  ( 109.9362594651775140, -2.948796715283049874, -6.904248079351286371 ) ) ;
#19310=CARTESIAN_POINT ( 'NONE',  ( 104.0571527818341906, -5.663308120860368611, -11.14355020191728762 ) ) ;
#19343=CARTESIAN_POINT ( 'NONE',  ( 129.3530333899765594, 6.000000000000000000, -57.49999999999999289 ) ) ;
#19365=CARTESIAN_POINT ( 'NONE',  ( -105.3347027237455080, 5.115232524641490919, 11.40545467192879947 ) ) ;
#19366=EDGE_CURVE ( 'NONE', #14308, #9458, #24614, .T. ) ;
#19368=EDGE_CURVE ( 'NONE', #24651, #6040, #20520, .T. ) ;
#19384=CARTESIAN_POINT ( 'NONE',  ( -101.6215955338914370, -3.854070255762961139, 6.439229133474693612 ) ) ;
#19427=DIRECTION ( 'NONE',  ( 0.000000000000000000, 0.000000000000000000, -1.000000000000000000 ) ) ;
#19429=CARTESIAN_POINT ( 'NONE',  ( 103.4583262007279245, 5.530333585247596773, 5.066783516361279993 ) ) ;
#19448=CARTESIAN_POINT ( 'NONE',  ( 105.0000000000000000, 0.000000000000000000, 60.00000000000000000 ) ) ;
#19458=DIRECTION ( 'NONE',  ( 0.000000000000000000, 0.000000000000000000, 1.000000000000000000 ) ) ;
#19481=ORIENTED_EDGE ( 'NONE', *, *, #11621, .T. ) ;
#19526=DIRECTION ( 'NONE',  ( -1.000000000000000000, -0.000000000000000000, -0.000000000000000000 ) ) ;
#19532=VECTOR ( 'NONE', #24676, 1000.000000000000000 ) ;
#19612=CARTESIAN_POINT ( 'NONE',  ( -99.95223371984603489, -0.8438318447813536460, -12.47259309357265522 ) ) ;
#19613=CIRCLE ( 'NONE', #24132, 5.738084889453667792 ) ;
#19666=CARTESIAN_POINT ( 'NONE',  ( 102.1109711573756016, -4.971563738489883200, -11.47098163371368251 ) ) ;
#19680=DIRECTION ( 'NONE',  ( -0.000000000000000000, -0.000000000000000000, 1.000000000000000000 ) ) ;
#19691=CARTESIAN_POINT ( 'NONE',  ( 99.26191511054632599, -4.118294838564020743E-16, -7.500000000000000000 ) ) ;
#19703=LINE ( 'NONE', #648, #9977 ) ;
#19769=CARTESIAN_POINT ( 'NONE',  ( -100.1500607241188021, -1.660053020383221778, 12.39330379916376224 ) ) ;
#19785=CARTESIAN_POINT ( 'NONE',  ( -99.92679314812558289, -0.6743631657302385785, -12.48293875069316528 ) ) ;
#19820=VERTEX_POINT ( 'NONE', #16781 ) ;
#19852=CARTESIAN_POINT ( 'NONE',  ( 99.26191511054634020, 0.3991779689724688773, -7.500000000000000000 ) ) ;
#19854=CONICAL_SURFACE ( 'NONE', #9018, 2.499999999999825473, 0.7853981633974538301 ) ;
#19856=EDGE_LOOP ( 'NONE', ( #17277, #22400 ) ) ;
#19871=CARTESIAN_POINT ( 'NONE',  ( 109.2847039433696779, -3.833500081834649187, -6.453260708061876905 ) ) ;
#19940=CARTESIAN_POINT ( 'NONE',  ( -100.0520116554321390, -1.339152422118498498, 12.43243648734289408 ) ) ;
#19956=CARTESIAN_POINT ( 'NONE',  ( -105.6714549178013840, -5.082150419746904291, -11.42046709103397895 ) ) ;
#20012=FACE_BOUND ( 'NONE', #1557, .T. ) ;
#20019=ORIENTED_EDGE ( 'NONE', *, *, #1990, .T. ) ;
#20025=DIRECTION ( 'NONE',  ( 0.000000000000000000, 0.000000000000000000, 1.000000000000000000 ) ) ;
#20119=CARTESIAN_POINT ( 'NONE',  ( -103.3398512556068738, -4.849606089681288701, 11.52174238786261107 ) ) ;
#20132=CARTESIAN_POINT ( 'NONE',  ( -100.6619007216472994, -2.715097909449887048, -12.20238416997437447 ) ) ;
#20164=VECTOR ( 'NONE', #12132, 1000.000000000000000 ) ;
#20170=EDGE_LOOP ( 'NONE', ( #34216, #20658, #23894, #16451 ) ) ;
#20175=CYLINDRICAL_SURFACE ( 'NONE', #28122, 10.00000000000000000 ) ;
#20181=ORIENTED_EDGE ( 'NONE', *, *, #28499, .T. ) ;
#20216=ORIENTED_EDGE ( 'NONE', *, *, #31503, .F. ) ;
#20281=CARTESIAN_POINT ( 'NONE',  ( 103.4967993190871169, 5.550581019792739212, 11.20035861729703086 ) ) ;
#20344=CARTESIAN_POINT ( 'NONE',  ( -105.0000000000000000, 0.000000000000000000, -57.49999999999999289 ) ) ;
#20401=ORIENTED_EDGE ( 'NONE', *, *, #30047, .T. ) ;
#20421=CARTESIAN_POINT ( 'NONE',  ( -109.0615761322723785, 3.126956236148902946, 12.10589691785418509 ) ) ;
#20432=CARTESIAN_POINT ( 'NONE',  ( 101.2097724487970964, -4.324042002361276005, 11.73155476838175559 ) ) ;
#20450=EDGE_LOOP ( 'NONE', ( #33372, #598, #11321, #13793 ) ) ;
#20452=CARTESIAN_POINT ( 'NONE',  ( 101.2030210553239726, 4.317991217963452755, 11.73376546078469040 ) ) ;
#20462=CARTESIAN_POINT ( 'NONE',  ( 129.3530333899765594, -6.000000000000000000, 62.49999999999999289 ) ) ;
#20493=ADVANCED_FACE ( 'NONE', ( #21137 ), #23454, .T. ) ;
#20514=LINE ( 'NONE', #31536, #33839 ) ;
#20520=LINE ( 'NONE', #4132, #7729 ) ;
#20525=PLANE ( 'NONE',  #21104 ) ;
#20537=CARTESIAN_POINT ( 'NONE',  ( 107.5878283054233293, 5.134660333356495521, -5.470525374126623319 ) ) ;
#20539=CARTESIAN_POINT ( 'NONE',  ( -110.1150203881707910, 3.829664765295703645E-16, -7.500000000000000000 ) ) ;
#20553=CONICAL_SURFACE ( 'NONE', #23391, 2.499999999999825473, 0.7853981633974538301 ) ;
#20557=ORIENTED_EDGE ( 'NONE', *, *, #27717, .T. ) ;
#20565=AXIS2_PLACEMENT_3D ( 'NONE', #12074, #11537, #25034 ) ;
#20600=CARTESIAN_POINT ( 'NONE',  ( 99.26191511054629757, -0.3789272201562040587, 12.50000000000000178 ) ) ;
#20603=CARTESIAN_POINT ( 'NONE',  ( 212.5000000000000000, 0.000000000000000000, 0.000000000000000000 ) ) ;
#20605=CARTESIAN_POINT ( 'NONE',  ( 129.3530333899765594, 6.000000000000000000, 62.49999999999999289 ) ) ;
#20634=FACE_OUTER_BOUND ( 'NONE', #16388, .T. ) ;
#20635=CARTESIAN_POINT ( 'NONE',  ( 129.3530333899765594, 6.000000000000000000, 57.49999999999999289 ) ) ;
#20647=CARTESIAN_POINT ( 'NONE',  ( 108.4960439411449897, -4.564063043377788453, 5.956988494001920209 ) ) ;
#20658=ORIENTED_EDGE ( 'NONE', *, *, #34359, .T. ) ;
#20666=EDGE_CURVE ( 'NONE', #16671, #20721, #1572, .T. ) ;
#20704=CYLINDRICAL_SURFACE ( 'NONE', #29046, 10.00000000000000000 ) ;
#20717=CARTESIAN_POINT ( 'NONE',  ( -108.3758620253048974, 3.856339488913134605, -6.437882550241565305 ) ) ;
#20721=VERTEX_POINT ( 'NONE', #34050 ) ;
#20722=CARTESIAN_POINT ( 'NONE',  ( 108.5065519622470021, 4.557154561855114139, -11.64184170122661932 ) ) ;
#20742=ORIENTED_EDGE ( 'NONE', *, *, #1524, .F. ) ;
#20774=CARTESIAN_POINT ( 'NONE',  ( 105.3748796498063030, -5.728975534391926416, 11.10987307012756631 ) ) ;
#20780=CARTESIAN_POINT ( 'NONE',  ( -110.1150203881707910, -0.3503014826537210746, -7.500000000000000888 ) ) ;
#20810=ORIENTED_EDGE ( 'NONE', *, *, #22356, .F. ) ;
#20819=CARTESIAN_POINT ( 'NONE',  ( 110.1062604042073474, -2.624171310066655938, 7.028111897042786715 ) ) ;
#20835=CARTESIAN_POINT ( 'NONE',  ( 105.0000000000000000, 0.000000000000000000, 60.00000000000000000 ) ) ;
#20843=CARTESIAN_POINT ( 'NONE',  ( -105.0000000000000000, 0.000000000000000000, 57.49999999999999289 ) ) ;
#20855=CARTESIAN_POINT ( 'NONE',  ( 109.5194798111833308, 3.554679846740550264, 6.612701241491620863 ) ) ;
#20882=CARTESIAN_POINT ( 'NONE',  ( 109.8329508816931366, 3.098707215121725422, -6.832002823648420708 ) ) ;
#20885=CARTESIAN_POINT ( 'NONE',  ( -109.4140444411644921, 2.605551551359102547, -7.039079951515507361 ) ) ;
#20890=CARTESIAN_POINT ( 'NONE',  ( 102.4416090844097482, 5.149687040066283750, -11.39104704602383933 ) ) ;
#20897=ORIENTED_EDGE ( 'NONE', *, *, #175, .F. ) ;
#20938=B_SPLINE_CURVE_WITH_KNOTS ( 'NONE', 3,
 ( #30741, #3501, #28249, #498, #14390, #846, #8498, #3676, #6342, #11892, #11711, #3848, #28067, #25390, #14742, #11182, #22739, #22032, #32874, #19365, #30206, #5809, #16705, #27537, #23428, #34285, #33938, #29116, #20421, #15261, #1374, #17592, #28600, #12066, #15087, #18120, #7215, #34105 ),
 .UNSPECIFIED., .F., .F.,
 ( 4, 2, 2, 2, 2, 2, 2, 2, 2, 2, 2, 2, 2, 2, 2, 2, 2, 2, 4 ),
 ( 1.577487858758373578E-18, 0.001010717872208361260, 0.002021435744416721220, 0.003032153616625081396, 0.004042871488833440705, 0.005053589361041800447, 0.006064307233250161057, 0.006569666169354321412, 0.007075025105458481768, 0.008085742977666759979, 0.009096460849875040791, 0.01010717872208332160, 0.01111789659429160242, 0.01212861446649988323, 0.01313933233870816578, 0.01364469127481231572, 0.01415005021091646741, 0.01516076808312478118, 0.01617148595533309322 ),
 .UNSPECIFIED. ) ;
#20961=CARTESIAN_POINT ( 'NONE',  ( 212.5000000000000000, 0.000000000000000000, 0.000000000000000000 ) ) ;
#20969=DIRECTION ( 'NONE',  ( -0.000000000000000000, -0.000000000000000000, -1.000000000000000000 ) ) ;
#20993=CARTESIAN_POINT ( 'NONE',  ( 104.0208154834590744, -5.657186516187210579, 4.924400946180165661 ) ) ;
#21029=CARTESIAN_POINT ( 'NONE',  ( 107.5863203406750870, 5.135442232304142429, 5.469792608531489186 ) ) ;
#21061=CARTESIAN_POINT ( 'NONE',  ( 109.9646280168875023, 2.883232572601705179, -12.16410353805738609 ) ) ;
#21070=ORIENTED_EDGE ( 'NONE', *, *, #8881, .F. ) ;
#21098=LINE ( 'NONE', #34455, #29148 ) ;
#21099=ORIENTED_EDGE ( 'NONE', *, *, #25588, .T. ) ;
#21104=AXIS2_PLACEMENT_3D ( 'NONE', #23205, #12354, #18397 ) ;
#21118=CARTESIAN_POINT ( 'NONE',  ( 108.7903099957938480, -4.324196401257810685, 11.73154709691606001 ) ) ;
#21127=DIRECTION ( 'NONE',  ( -0.000000000000000000, 0.000000000000000000, -1.000000000000000000 ) ) ;
#21137=FACE_OUTER_BOUND ( 'NONE', #23483, .T. ) ;
#21142=VECTOR ( 'NONE', #9253, 1000.000000000000000 ) ;
#21168=CARTESIAN_POINT ( 'NONE',  ( 105.7855116681631245, -5.687452395779748038, 4.889156772952023999 ) ) ;
#21206=DIRECTION ( 'NONE',  ( 0.000000000000000000, 0.000000000000000000, -1.000000000000000000 ) ) ;
#21220=VECTOR ( 'NONE', #29950, 1000.000000000000000 ) ;
#21232=CARTESIAN_POINT ( 'NONE',  ( 110.7380848894536740, 0.3953117532656757471, -7.500000000000019540 ) ) ;
#21237=VERTEX_POINT ( 'NONE', #7975 ) ;
#21300=CARTESIAN_POINT ( 'NONE',  ( -99.88497961182919482, -2.585407550593147656E-15, 7.500000000000000000 ) ) ;
#21332=CARTESIAN_POINT ( 'NONE',  ( -108.3810596861186610, 3.852356953585670318, -11.89405885704114141 ) ) ;
#21353=CARTESIAN_POINT ( 'NONE',  ( 99.58179902723867372, -1.926730348087509981, 7.257477599627513598 ) ) ;
#21391=CARTESIAN_POINT ( 'NONE',  ( 108.4949890547536455, 4.564908081027950537, 5.956352141036524550 ) ) ;
#21410=DIRECTION ( 'NONE',  ( -1.000000000000000000, -0.000000000000000000, -0.000000000000000000 ) ) ;
#21423=CARTESIAN_POINT ( 'NONE',  ( 104.2390490158698526, 5.700015625666662089, -11.12505441474362478 ) ) ;
#21469=PLANE ( 'NONE',  #10322 ) ;
#21476=CARTESIAN_POINT ( 'NONE',  ( -105.6885685459855893, 5.080227507390848274, 5.518150456212836730 ) ) ;
#21481=CARTESIAN_POINT ( 'NONE',  ( -109.7700750224988582, -1.854090048725078432, -7.268955362025010025 ) ) ;
#21505=CARTESIAN_POINT ( 'NONE',  ( -100.6601417511032395, 2.712336548677835246, -12.20300697856195882 ) ) ;
#21508=VECTOR ( 'NONE', #6764, 1000.000000000000000 ) ;
#21581=ORIENTED_EDGE ( 'NONE', *, *, #13680, .F. ) ;
#21586=ADVANCED_FACE ( 'NONE', ( #4091 ), #28672, .T. ) ;
#21591=CARTESIAN_POINT ( 'NONE',  ( -99.88497961182919482, 6.264093345946821604E-16, 60.00000000000000000 ) ) ;
#21596=CARTESIAN_POINT ( 'NONE',  ( 110.7380848894537166, -0.1972643383979439669, -7.500000000000013323 ) ) ;
#21597=AXIS2_PLACEMENT_3D ( 'NONE', #20344, #15006, #6620 ) ;
#21616=CARTESIAN_POINT ( 'NONE',  ( 107.5565492092080859, -5.150622582557323526, -11.39062369188951251 ) ) ;
#21619=LINE ( 'NONE', #18788, #7711 ) ;
#21636=ORIENTED_EDGE ( 'NONE', *, *, #1524, .T. ) ;
#21669=CARTESIAN_POINT ( 'NONE',  ( -106.3376375495021335, 4.939893293632461990, -11.48260997023825958 ) ) ;
#21687=CARTESIAN_POINT ( 'NONE',  ( -109.3194926363487269, -2.744499711777497186, 6.981349484866706590 ) ) ;
#21751=CARTESIAN_POINT ( 'NONE',  ( -130.6469666100234406, -6.000000000000000000, 62.49999999999999289 ) ) ;
#21774=LINE ( 'NONE', #21956, #19033 ) ;
#21785=CARTESIAN_POINT ( 'NONE',  ( 110.2200992156835042, -2.389942209051219457, -12.27067588826158939 ) ) ;
#21801=CARTESIAN_POINT ( 'NONE',  ( -130.6469666100234406, -6.000000000000000000, -57.49999999999999289 ) ) ;
#21814=CARTESIAN_POINT ( 'NONE',  ( -101.6241379746951452, 3.856339488913145264, 6.437882550241559976 ) ) ;
#21841=CARTESIAN_POINT ( 'NONE',  ( -101.6156648126628568, 3.849558703864950804, -11.89498339909459723 ) ) ;
#21864=CARTESIAN_POINT ( 'NONE',  ( -110.1062952961228376, -0.3451077285824886154, 7.494041212912380345 ) ) ;
#21871=DIRECTION ( 'NONE',  ( 0.000000000000000000, 0.000000000000000000, 1.000000000000000000 ) ) ;
#21880=AXIS2_PLACEMENT_3D ( 'NONE', #2287, #7806, #16019 ) ;
#21933=AXIS2_PLACEMENT_3D ( 'NONE', #30828, #28339, #11623 ) ;
#21956=CARTESIAN_POINT ( 'NONE',  ( -117.4999999999997442, 0.000000000000000000, -12.50000000000000000 ) ) ;
#21963=FACE_OUTER_BOUND ( 'NONE', #34123, .T. ) ;
#21968=CARTESIAN_POINT ( 'NONE',  ( -117.4999999999997442, 0.000000000000000000, 0.000000000000000000 ) ) ;
#21970=CARTESIAN_POINT ( 'NONE',  ( 105.3825092702455777, -5.728493955922442815, -11.11012212270734167 ) ) ;
#21995=PRODUCT_DEFINITION_SHAPE ( 'NONE', 'NONE',  #25992 ) ;
#22001=CARTESIAN_POINT ( 'NONE',  ( -100.4259553087715204, 2.313922778582933937, 7.141321738367093275 ) ) ;
#22006=ADVANCED_BREP_SHAPE_REPRESENTATION ( '', ( #34055, #28566 ), #32533 ) ;
#22014=CARTESIAN_POINT ( 'NONE',  ( 117.4999999999998579, 0.000000000000000000, 0.000000000000000000 ) ) ;
#22032=CARTESIAN_POINT ( 'NONE',  ( -104.3244124248265052, 5.081434799294422433, 11.42078282599712935 ) ) ;
#22049=CARTESIAN_POINT ( 'NONE',  ( 110.6956932917700271, -0.7984011589207654636, 7.467432841349395112 ) ) ;
#22110=AXIS2_PLACEMENT_3D ( 'NONE', #16345, #32506, #29675 ) ;
#22175=FACE_OUTER_BOUND ( 'NONE', #4746, .T. ) ;
#22222=CARTESIAN_POINT ( 'NONE',  ( -100.1713109292253705, -1.696008709688489047, 7.307621933264760727 ) ) ;
#22265=CARTESIAN_POINT ( 'NONE',  ( 99.30232950514738377, 0.7843626702862538380, 7.468944954497490407 ) ) ;
#22271=CARTESIAN_POINT ( 'NONE',  ( -106.6601487443931262, -4.849606089681288701, -11.52174238786261107 ) ) ;
#22286=PRODUCT ( 'shaft', 'shaft', '', ( #8201 ) ) ;
#22293=FACE_OUTER_BOUND ( 'NONE', #10718, .T. ) ;
#22308=ORIENTED_EDGE ( 'NONE', *, *, #14194, .T. ) ;
#22323=DIRECTION ( 'NONE',  ( 0.000000000000000000, 0.000000000000000000, 1.000000000000000000 ) ) ;
#22336=ADVANCED_FACE ( 'NONE', ( #8980 ), #6286, .T. ) ;
#22356=EDGE_CURVE ( 'NONE', #16360, #25686, #22919, .T. ) ;
#22360=ORIENTED_EDGE ( 'NONE', *, *, #6425, .T. ) ;
#22400=ORIENTED_EDGE ( 'NONE', *, *, #10323, .T. ) ;
#22407=DIRECTION ( 'NONE',  ( -0.000000000000000000, -0.000000000000000000, -1.000000000000000000 ) ) ;
#22440=VECTOR ( 'NONE', #12093, 1000.000000000000000 ) ;
#22445=CARTESIAN_POINT ( 'NONE',  ( 99.58837370945708756, 1.917593826231215770, 7.253178031220425481 ) ) ;
#22488=ORIENTED_EDGE ( 'NONE', *, *, #26308, .T. ) ;
#22496=ORIENTED_EDGE ( 'NONE', *, *, #7135, .F. ) ;
#22520=B_SPLINE_CURVE_WITH_KNOTS ( 'NONE', 3,
 ( #20539, #9850, #18405, #4661, #31898, #4148, #20885, #7516, #1837, #20717, #2017, #31563, #15553, #34765, #26396, #15039, #23554, #31393, #12717, #28723, #12893, #6997, #4322, #15209, #26052, #2712, #5717, #24776, #16619, #29428, #3061, #7881, #5544, #24416, #32784, #24245 ),
 .UNSPECIFIED., .F., .F.,
 ( 4, 2, 2, 2, 2, 2, 2, 2, 2, 2, 2, 2, 2, 2, 2, 2, 2, 4 ),
 ( 3.708067775211463633E-19, 0.001035696236907465012, 0.002071392473814929591, 0.003107088710722395036, 0.004142784947629859181, 0.005178481184537325061, 0.006214177421444790073, 0.007249873658352254217, 0.007767721776805967641, 0.008285569895259680198, 0.009321266132167145210, 0.01035696236907461369, 0.01087481048752832885, 0.01139265860598204401, 0.01242835484288950555, 0.01449974731670440609, 0.01553544355361185722, 0.01657113979051930489 ),
 .UNSPECIFIED. ) ;
#22524=AXIS2_PLACEMENT_3D ( 'NONE', #1097, #20969, #17318 ) ;
#22529=ORIENTED_EDGE ( 'NONE', *, *, #29437, .F. ) ;
#22541=ORIENTED_EDGE ( 'NONE', *, *, #28121, .F. ) ;
#22583=ORIENTED_EDGE ( 'NONE', *, *, #14193, .F. ) ;
#22607=DIRECTION ( 'NONE',  ( -0.000000000000000000, -0.000000000000000000, -1.000000000000000000 ) ) ;
#22612=CARTESIAN_POINT ( 'NONE',  ( -109.5827309310070916, -2.278159677709880704, 12.29156386665007084 ) ) ;
#22630=CARTESIAN_POINT ( 'NONE',  ( -102.7235731336728719, -4.592708079286355272, -11.62653478258734907 ) ) ;
#22697=DIRECTION ( 'NONE',  ( -1.000000000000000000, -0.000000000000000000, -0.000000000000000000 ) ) ;
#22703=DIRECTION ( 'NONE',  ( 0.000000000000000000, 0.000000000000000000, -1.000000000000000000 ) ) ;
#22716=ORIENTED_EDGE ( 'NONE', *, *, #29545, .F. ) ;
#22724=DIRECTION ( 'NONE',  ( -0.000000000000000000, -0.000000000000000000, -1.000000000000000000 ) ) ;
#22727=CARTESIAN_POINT ( 'NONE',  ( 129.3530333899765594, -6.000000000000000000, -62.49999999999999289 ) ) ;
#22729=CIRCLE ( 'NONE', #21597, 5.115020388170798959 ) ;
#22735=CARTESIAN_POINT ( 'NONE',  ( -130.6469666100234406, 6.000000000000000000, 62.49999999999999289 ) ) ;
#22736=EDGE_LOOP ( 'NONE', ( #9868, #27467 ) ) ;
#22739=CARTESIAN_POINT ( 'NONE',  ( -103.8279344131445470, 4.981785521925213622, 11.46442881298733241 ) ) ;
#22747=VECTOR ( 'NONE', #23998, 1000.000000000000000 ) ;
#22769=CARTESIAN_POINT ( 'NONE',  ( 106.8660777065885412, 5.429478283318180054, 11.25942253076638089 ) ) ;
#22774=FACE_OUTER_BOUND ( 'NONE', #29218, .T. ) ;
#22780=CARTESIAN_POINT ( 'NONE',  ( -109.9476998985492173, -1.340877102867428894, 12.43231962408541769 ) ) ;
#22797=CARTESIAN_POINT ( 'NONE',  ( -100.1505957388136494, -1.661087400543260761, -12.39310421627767944 ) ) ;
#22828=SHAPE_REPRESENTATION_RELATIONSHIP ( 'NONE' , 'NONE' ,  #18474, #22006 ) ;
#22839=DIRECTION ( 'NONE',  ( 0.000000000000000000, 0.000000000000000000, 1.000000000000000000 ) ) ;
#22884=CARTESIAN_POINT ( 'NONE',  ( 107.8989562062458560, -4.964839546134684589, -5.627339305134570147 ) ) ;
#22919=CIRCLE ( 'NONE', #9268, 10.00000000000000000 ) ;
#22922=VERTEX_POINT ( 'NONE', #16748 ) ;
#22944=CARTESIAN_POINT ( 'NONE',  ( 107.8850264453569707, 4.974089543361914778, 11.46991629550682212 ) ) ;
#22951=ORIENTED_EDGE ( 'NONE', *, *, #26103, .T. ) ;
#22971=CARTESIAN_POINT ( 'NONE',  ( -109.8499392758812121, -1.660053020383221112, -12.39330379916376756 ) ) ;
#23030=FACE_BOUND ( 'NONE', #9308, .T. ) ;
#23099=VERTEX_POINT ( 'NONE', #1415 ) ;
#23105=CARTESIAN_POINT ( 'NONE',  ( 110.7380848894537024, -0.3844778738587160682, 12.50000000000000178 ) ) ;
#23130=CARTESIAN_POINT ( 'NONE',  ( 110.5504696841441046, 1.503590720865120911, 12.41481623251361555 ) ) ;
#23148=EDGE_CURVE ( 'NONE', #10220, #9458, #17995, .T. ) ;
#23205=CARTESIAN_POINT ( 'NONE',  ( 0.000000000000000000, 0.000000000000000000, -57.49999999999999289 ) ) ;
#23212=DIRECTION ( 'NONE',  ( -1.000000000000000000, 0.000000000000000000, 0.000000000000000000 ) ) ;
#23225=EDGE_LOOP ( 'NONE', ( #9260, #30276, #20810, #31046 ) ) ;
#23232=CARTESIAN_POINT ( 'NONE',  ( 100.4809210094639980, -3.554721378204152682, -6.612463615769124559 ) ) ;
#23241=CARTESIAN_POINT ( 'NONE',  ( 129.3530333899765594, 6.000000000000000000, -62.49999999999999289 ) ) ;
#23277=CARTESIAN_POINT ( 'NONE',  ( 110.6987342991635188, -0.7699128213881768490, 12.48180554319666768 ) ) ;
#23282=DIRECTION ( 'NONE',  ( 1.000000000000000000, 0.000000000000000000, -0.000000000000000000 ) ) ;
#23297=EDGE_CURVE ( 'NONE', #8267, #6040, #20938, .T. ) ;
#23320=CARTESIAN_POINT ( 'NONE',  ( -110.1150203881707910, -7.176976838982289656E-16, -12.50000000000000000 ) ) ;
#23344=ORIENTED_EDGE ( 'NONE', *, *, #11983, .F. ) ;
#23375=CARTESIAN_POINT ( 'NONE',  ( 110.1953605866412715, 2.443267496989373733, -7.093208238637026319 ) ) ;
#23384=CARTESIAN_POINT ( 'NONE',  ( 109.3193400707606031, 3.795444455902927228, -11.91305592319909223 ) ) ;
#23391=AXIS2_PLACEMENT_3D ( 'NONE', #7676, #13044, #18572 ) ;
#23424=ORIENTED_EDGE ( 'NONE', *, *, #25270, .T. ) ;
#23428=CARTESIAN_POINT ( 'NONE',  ( -107.5740197209480726, 4.432569708812558851, 11.68934771181378451 ) ) ;
#23439=CARTESIAN_POINT ( 'NONE',  ( 104.6174907297543939, -5.728493955922441927, 11.11012212270733990 ) ) ;
#23454=PLANE ( 'NONE',  #4372 ) ;
#23481=CARTESIAN_POINT ( 'NONE',  ( 109.8288047610148936, -3.105058450138034498, 6.829076936735990699 ) ) ;
#23483=EDGE_LOOP ( 'NONE', ( #32489, #16495, #20557, #27558 ) ) ;
#23523=CARTESIAN_POINT ( 'NONE',  ( 110.1195297133390625, 2.618976401886136340, 7.037310091161540271 ) ) ;
#23550=DIRECTION ( 'NONE',  ( -1.000000000000000000, 0.000000000000000000, 0.000000000000000000 ) ) ;
#23554=CARTESIAN_POINT ( 'NONE',  ( -105.6968603966071498, 5.070301591678565423, -5.526538532257564640 ) ) ;
#23559=CARTESIAN_POINT ( 'NONE',  ( 99.56251466041456410, 1.870982065537967420, -12.36420004006153839 ) ) ;
#23619=CARTESIAN_POINT ( 'NONE',  ( 109.9600497711273448, -2.891119662789794820, 12.16223328578254836 ) ) ;
#23626=CARTESIAN_POINT ( 'NONE',  ( -101.6279274993559198, -3.859727759966185001, -6.435874498883202399 ) ) ;
#23662=CARTESIAN_POINT ( 'NONE',  ( 102.1010437937541298, -4.964839546134684589, 5.627339305134570147 ) ) ;
#23686=EDGE_CURVE ( 'NONE', #21237, #16, #7457, .T. ) ;
#23702=CARTESIAN_POINT ( 'NONE',  ( 107.9015628886182867, 4.963291960430601613, 5.628698742319545367 ) ) ;
#23718=DIRECTION ( 'NONE',  ( -0.000000000000000000, -0.000000000000000000, -1.000000000000000000 ) ) ;
#23719=EDGE_CURVE ( 'NONE', #6202, #24651, #14304, .T. ) ;
#23780=ORIENTED_EDGE ( 'NONE', *, *, #27361, .F. ) ;
#23793=CARTESIAN_POINT ( 'NONE',  ( 105.9428472181658236, -5.663308120860370387, 11.14355020191728940 ) ) ;
#23795=FACE_BOUND ( 'NONE', #22736, .T. ) ;
#23806=DIRECTION ( 'NONE',  ( 0.000000000000000000, 0.000000000000000000, 1.000000000000000000 ) ) ;
#23808=CARTESIAN_POINT ( 'NONE',  ( 99.26191511054632599, 0.000000000000000000, -57.49999999999999289 ) ) ;
#23814=CARTESIAN_POINT ( 'NONE',  ( 99.26191511054632599, 1.643815732525060864E-21, 12.50000000000000000 ) ) ;
#23837=LINE ( 'NONE', #32198, #22747 ) ;
#23876=CARTESIAN_POINT ( 'NONE',  ( 127.4999999999999147, 0.000000000000000000, 0.000000000000000000 ) ) ;
#23890=CARTESIAN_POINT ( 'NONE',  ( 110.5782799041639350, 1.358924363732619600, -7.378408734721662476 ) ) ;
#23894=ORIENTED_EDGE ( 'NONE', *, *, #7789, .F. ) ;
#23928=ORIENTED_EDGE ( 'NONE', *, *, #13680, .T. ) ;
#23931=EDGE_CURVE ( 'NONE', #6040, #8267, #10273, .T. ) ;
#23935=DIRECTION ( 'NONE',  ( -1.000000000000000000, -0.000000000000000000, -0.000000000000000000 ) ) ;
#23957=CARTESIAN_POINT ( 'NONE',  ( -99.88497961182919482, 9.184690493976639608E-16, -7.500000000000000000 ) ) ;
#23963=CARTESIAN_POINT ( 'NONE',  ( -130.6469666100234406, 6.000000000000000000, 62.49999999999999289 ) ) ;
#23998=DIRECTION ( 'NONE',  ( 1.000000000000000000, 0.000000000000000000, 0.000000000000000000 ) ) ;
#24036=CARTESIAN_POINT ( 'NONE',  ( 110.4189565558304906, 1.924456215511286983, 7.258046499395033102 ) ) ;
#24038=EDGE_CURVE ( 'NONE', #25686, #16360, #12018, .T. ) ;
#24089=ORIENTED_EDGE ( 'NONE', *, *, #9336, .F. ) ;
#24092=ADVANCED_FACE ( 'NONE', ( #15836 ), #26667, .T. ) ;
#24093=DIRECTION ( 'NONE',  ( -1.000000000000000000, 0.000000000000000000, -0.000000000000000000 ) ) ;
#24106=CYLINDRICAL_SURFACE ( 'NONE', #8076, 7.500000000000000000 ) ;
#24129=CARTESIAN_POINT ( 'NONE',  ( -107.1458265010192861, 4.646131333787441697, 5.888157618374225244 ) ) ;
#24132=AXIS2_PLACEMENT_3D ( 'NONE', #27903, #27205, #30059 ) ;
#24134=CARTESIAN_POINT ( 'NONE',  ( -109.4154700880919080, -2.602876666701938291, -7.039998176148507092 ) ) ;
#24139=CARTESIAN_POINT ( 'NONE',  ( 127.4999999999999147, 0.000000000000000000, 12.50000000000000000 ) ) ;
#24160=CARTESIAN_POINT ( 'NONE',  ( -106.6598137192883939, 4.841160850826504713, -11.52458411820204454 ) ) ;
#24170=VECTOR ( 'NONE', #13647, 1000.000000000000000 ) ;
#24245=CARTESIAN_POINT ( 'NONE',  ( -99.88497961182919482, 9.184690493976639608E-16, -7.500000000000000000 ) ) ;
#24304=EDGE_CURVE ( 'NONE', #7139, #14417, #24528, .T. ) ;
#24307=CARTESIAN_POINT ( 'NONE',  ( -109.9748806441469924, -1.201525761660785951, -7.405089084531744525 ) ) ;
#24336=CARTESIAN_POINT ( 'NONE',  ( 127.4999999999999147, 1.530808498934191521E-15, -12.50000000000000000 ) ) ;
#24351=CARTESIAN_POINT ( 'NONE',  ( -110.1150203881707910, -1.604996202923496961E-20, 7.500000000000000000 ) ) ;
#24416=CARTESIAN_POINT ( 'NONE',  ( -99.92113738465764072, 0.6978363313042835747, -7.475210363867073937 ) ) ;
#24431=DIRECTION ( 'NONE',  ( -0.000000000000000000, -0.000000000000000000, -1.000000000000000000 ) ) ;
#24466=CARTESIAN_POINT ( 'NONE',  ( -100.0586838875211413, 1.365406536427365758, 7.382450522560827899 ) ) ;
#24496=CARTESIAN_POINT ( 'NONE',  ( -102.4259802790519416, 4.432569708812561515, -11.68934771181378629 ) ) ;
#24501=ORIENTED_EDGE ( 'NONE', *, *, #11144, .F. ) ;
#24505=DIRECTION ( 'NONE',  ( -1.000000000000000000, -0.000000000000000000, -0.000000000000000000 ) ) ;
#24528=CIRCLE ( 'NONE', #20565, 10.00000000000000000 ) ;
#24561=CARTESIAN_POINT ( 'NONE',  ( 99.26191511054601335, -2.804307960831458189E-14, 7.500000000000241585 ) ) ;
#24587=LINE ( 'NONE', #18760, #21220 ) ;
#24596=ORIENTED_EDGE ( 'NONE', *, *, #6057, .T. ) ;
#24614=LINE ( 'NONE', #8433, #28754 ) ;
#24616=DIRECTION ( 'NONE',  ( 1.000000000000000000, -0.000000000000000000, -0.000000000000000000 ) ) ;
#24650=CARTESIAN_POINT ( 'NONE',  ( -109.0659643713068903, 3.171022835462813383, 6.816853140736490069 ) ) ;
#24651=VERTEX_POINT ( 'NONE', #15966 ) ;
#24676=DIRECTION ( 'NONE',  ( -1.000000000000000000, -0.000000000000000000, -0.000000000000000000 ) ) ;
#24680=CARTESIAN_POINT ( 'NONE',  ( -100.0523128185887600, 1.341502966352551951, -12.43231302123709625 ) ) ;
#24702=CARTESIAN_POINT ( 'NONE',  ( -106.3650732166412638, -4.941537997685736094, 5.642681918066573488 ) ) ;
#24748=CARTESIAN_POINT ( 'NONE',  ( 104.0203572285688267, 5.657131480001861057, 4.924467467246998353 ) ) ;
#24772=DIRECTION ( 'NONE',  ( -1.000000000000000000, 0.000000000000000000, 0.000000000000000000 ) ) ;
#24776=CARTESIAN_POINT ( 'NONE',  ( -101.8759042855232479, 4.062957613056754624, -6.307943406627036786 ) ) ;
#24833=CARTESIAN_POINT ( 'NONE',  ( 129.3530333899765594, 6.000000000000000000, 57.49999999999999289 ) ) ;
#24879=CARTESIAN_POINT ( 'NONE',  ( -100.5845299119079925, -2.602876666701936514, 7.039998176148507980 ) ) ;
#24940=DIRECTION ( 'NONE',  ( -0.000000000000000000, -0.000000000000000000, -1.000000000000000000 ) ) ;
#24945=DIRECTION ( 'NONE',  ( -1.000000000000000000, 0.000000000000000000, 0.000000000000000000 ) ) ;
#24973=CARTESIAN_POINT ( 'NONE',  ( 105.0034891410423512, -5.747432938596947594, -11.10030587185099726 ) ) ;
#24978=CYLINDRICAL_SURFACE ( 'NONE', #2785, 5.115020388170798959 ) ;
#24990=CARTESIAN_POINT ( 'NONE',  ( -105.0000000000000000, 0.000000000000000000, 57.49999999999999289 ) ) ;
#25034=DIRECTION ( 'NONE',  ( 0.000000000000000000, 0.000000000000000000, -1.000000000000000000 ) ) ;
#25035=CARTESIAN_POINT ( 'NONE',  ( -119.9999999999997726, 0.000000000000000000, 0.000000000000000000 ) ) ;
#25056=CYLINDRICAL_SURFACE ( 'NONE', #5949, 5.738084889453667792 ) ;
#25077=CARTESIAN_POINT ( 'NONE',  ( -110.1067333817248226, -0.3368495349214609136, 12.49660185505138976 ) ) ;
#25088=EDGE_CURVE ( 'NONE', #11373, #1125, #17417, .T. ) ;
#25093=CARTESIAN_POINT ( 'NONE',  ( 106.5405508486335293, 5.530628908288163004, 5.066456342206738128 ) ) ;
#25098=CARTESIAN_POINT ( 'NONE',  ( -110.1150203881707483, -0.3417625387765728107, -12.49999999999999822 ) ) ;
#25107=ORIENTED_EDGE ( 'NONE', *, *, #35084, .F. ) ;
#25152=CARTESIAN_POINT ( 'NONE',  ( 108.5055490898496373, -4.557852096327890123, -11.64155778436300182 ) ) ;
#25246=CARTESIAN_POINT ( 'NONE',  ( 107.5583909155902802, 5.149687040066284638, 11.39104704602384466 ) ) ;
#25254=DIRECTION ( 'NONE',  ( -1.000000000000000000, 0.000000000000000000, 0.000000000000000000 ) ) ;
#25261=CARTESIAN_POINT ( 'NONE',  ( -106.3407376400858055, -4.947629808455843659, 11.47938275244241524 ) ) ;
#25264=EDGE_CURVE ( 'NONE', #17516, #19142, #18627, .T. ) ;
#25270=EDGE_CURVE ( 'NONE', #3925, #17170, #21098, .T. ) ;
#25274=DIRECTION ( 'NONE',  ( 0.7071067811865512365, 0.000000000000000000, -0.7071067811865439090 ) ) ;
#25279=EDGE_LOOP ( 'NONE', ( #26965, #15079, #8419, #3568, #26186, #17994, #28664, #18815, #11898, #16958, #26786, #27394 ) ) ;
#25342=CARTESIAN_POINT ( 'NONE',  ( 99.46174900952425446, 1.550744593849150865, -7.348056298371736794 ) ) ;
#25351=DIRECTION ( 'NONE',  ( 1.000000000000000000, -0.000000000000000000, -0.000000000000000000 ) ) ;
#25390=CARTESIAN_POINT ( 'NONE',  ( -103.1830246108492162, 4.784316299155410235, 11.54838096230724176 ) ) ;
#25406=CARTESIAN_POINT ( 'NONE',  ( -110.1150203881707910, -7.176976838982289656E-16, -12.50000000000000000 ) ) ;
#25407=DIRECTION ( 'NONE',  ( -0.000000000000000000, -0.000000000000000000, 1.000000000000000000 ) ) ;
#25439=CARTESIAN_POINT ( 'NONE',  ( -101.6198087930189757, -3.853301823223607592, 11.89378582241138993 ) ) ;
#25443=VECTOR ( 'NONE', #29910, 1000.000000000000000 ) ;
#25465=CARTESIAN_POINT ( 'NONE',  ( 129.3530333899765594, 6.000000000000000000, 62.49999999999999289 ) ) ;
#25495=DIRECTION ( 'NONE',  ( -0.000000000000000000, 1.000000000000000000, -0.000000000000000000 ) ) ;
#25519=CARTESIAN_POINT ( 'NONE',  ( 103.6432141880921876, 5.578687132273540961, -5.013157219915588492 ) ) ;
#25535=CARTESIAN_POINT ( 'NONE',  ( 105.3932757502030881, -5.728011724833245388, -4.841576811596270069 ) ) ;
#25537=ORIENTED_EDGE ( 'NONE', *, *, #13618, .T. ) ;
#25580=DIRECTION ( 'NONE',  ( 0.000000000000000000, 0.000000000000000000, 1.000000000000000000 ) ) ;
#25588=EDGE_CURVE ( 'NONE', #13528, #14561, #11477, .T. ) ;
#25612=CARTESIAN_POINT ( 'NONE',  ( -100.4106824525208168, -2.283823867687215348, 12.29365298152801955 ) ) ;
#25627=CARTESIAN_POINT ( 'NONE',  ( -109.1548934309756049, -2.987912174852651148, -12.13846169321889512 ) ) ;
#25673=CARTESIAN_POINT ( 'NONE',  ( 212.5000000000000000, 0.000000000000000000, 0.000000000000000000 ) ) ;
#25674=ORIENTED_EDGE ( 'NONE', *, *, #23148, .T. ) ;
#25680=EDGE_CURVE ( 'NONE', #33855, #9756, #24587, .T. ) ;
#25686=VERTEX_POINT ( 'NONE', #13236 ) ;
#25698=CARTESIAN_POINT ( 'NONE',  ( 102.9230630902097374, 5.352195967840122748, -5.254935570228769670 ) ) ;
#25700=DIRECTION ( 'NONE',  ( 0.000000000000000000, 0.000000000000000000, 1.000000000000000000 ) ) ;
#25748=EDGE_CURVE ( 'NONE', #6202, #8267, #5190, .T. ) ;
#25757=CARTESIAN_POINT ( 'NONE',  ( -130.6469666100234406, -6.000000000000000000, -62.49999999999999289 ) ) ;
#25777=ORIENTED_EDGE ( 'NONE', *, *, #34359, .F. ) ;
#25791=CARTESIAN_POINT ( 'NONE',  ( -100.5687310144427045, -2.576157761670764934, 12.23490486094944174 ) ) ;
#25817=VECTOR ( 'NONE', #27813, 1000.000000000000000 ) ;
#25909=DIRECTION ( 'NONE',  ( -0.000000000000000000, -0.000000000000000000, -1.000000000000000000 ) ) ;
#25939=CARTESIAN_POINT ( 'NONE',  ( 101.4944509101503911, -4.557852096327890123, 11.64155778436300182 ) ) ;
#25958=EDGE_LOOP ( 'NONE', ( #23928, #19481 ) ) ;
#25961=CARTESIAN_POINT ( 'NONE',  ( 100.1328585621623120, 3.044914778013036116, 12.12453154756074802 ) ) ;
#25986=LINE ( 'NONE', #26332, #20164 ) ;
#25992=PRODUCT_DEFINITION ( 'UNKNOWN', '', #33179, #26712 ) ;
#26022=FACE_OUTER_BOUND ( 'NONE', #23225, .T. ) ;
#26052=CARTESIAN_POINT ( 'NONE',  ( -102.7041492557062128, 4.573766672917669140, -5.944761500833685375 ) ) ;
#26056=CARTESIAN_POINT ( 'NONE',  ( 110.7380848894536456, 0.3793982372081800558, -12.50000000000000178 ) ) ;
#26073=LINE ( 'NONE', #23241, #4587 ) ;
#26103=EDGE_CURVE ( 'NONE', #20721, #19820, #29017, .T. ) ;
#26109=CARTESIAN_POINT ( 'NONE',  ( 104.0474366975612526, -5.661646449284259752, 11.14439484353663090 ) ) ;
#26140=EDGE_LOOP ( 'NONE', ( #6159, #13426, #22951, #14619 ) ) ;
#26156=EDGE_LOOP ( 'NONE', ( #8392, #8160, #24596, #6015 ) ) ;
#26186=ORIENTED_EDGE ( 'NONE', *, *, #31503, .T. ) ;
#26188=ORIENTED_EDGE ( 'NONE', *, *, #10253, .T. ) ;
#26212=CARTESIAN_POINT ( 'NONE',  ( 110.4116262905429267, 1.917593826231215770, -7.253178031220425481 ) ) ;
#26221=CARTESIAN_POINT ( 'NONE',  ( 105.7593996005910100, 5.690832488206153172, -11.12946004024182756 ) ) ;
#26281=CARTESIAN_POINT ( 'NONE',  ( 108.5044842081497194, -4.558675695222540902, 11.64123453730966595 ) ) ;
#26300=VECTOR ( 'NONE', #28244, 1000.000000000000000 ) ;
#26308=EDGE_CURVE ( 'NONE', #16671, #30104, #33627, .T. ) ;
#26332=CARTESIAN_POINT ( 'NONE',  ( 99.26191511054632599, 0.000000000000000000, 60.00000000000000000 ) ) ;
#26366=CARTESIAN_POINT ( 'NONE',  ( 108.7751028178685431, 4.336304859840375059, 6.126759150192703451 ) ) ;
#26375=DIRECTION ( 'NONE',  ( 0.000000000000000000, 0.000000000000000000, -1.000000000000000000 ) ) ;
#26396=CARTESIAN_POINT ( 'NONE',  ( -106.3672936988086235, 4.940661300061105266, -5.643441299694564428 ) ) ;
#26401=CARTESIAN_POINT ( 'NONE',  ( 99.26191511054632599, -6.978196330887525654E-16, -12.50000000000000000 ) ) ;
#26411=ORIENTED_EDGE ( 'NONE', *, *, #11144, .T. ) ;
#26479=CARTESIAN_POINT ( 'NONE',  ( 117.4999999999998579, 1.530808498934191521E-15, -12.50000000000000000 ) ) ;
#26496=VERTEX_POINT ( 'NONE', #1239 ) ;
#26514=VERTEX_POINT ( 'NONE', #33807 ) ;
#26579=CARTESIAN_POINT ( 'NONE',  ( 0.000000000000000000, 0.000000000000000000, 0.000000000000000000 ) ) ;
#26599=FACE_OUTER_BOUND ( 'NONE', #30584, .T. ) ;
#26633=CARTESIAN_POINT ( 'NONE',  ( 110.7380848894536598, 7.027127293105233764E-16, 12.50000000000000000 ) ) ;
#26636=DIRECTION ( 'NONE',  ( 1.000000000000000000, 0.000000000000000000, 0.000000000000000000 ) ) ;
#26639=CARTESIAN_POINT ( 'NONE',  ( -100.1618820091562014, -1.694081942180570177, -7.313267332261218279 ) ) ;
#26643=EDGE_LOOP ( 'NONE', ( #13403, #16834, #33786, #20742 ) ) ;
#26645=ORIENTED_EDGE ( 'NONE', *, *, #25270, .F. ) ;
#26667=CYLINDRICAL_SURFACE ( 'NONE', #30779, 10.00000000000000000 ) ;
#26712=PRODUCT_DEFINITION_CONTEXT ( 'detailed design', #9642, 'design' ) ;
#26741=CARTESIAN_POINT ( 'NONE',  ( -262.5000000000000000, 0.000000000000000000, 0.000000000000000000 ) ) ;
#26750=CARTESIAN_POINT ( 'NONE',  ( 100.3425380856783278, 3.356865266134898995, -12.04189187465341782 ) ) ;
#26786=ORIENTED_EDGE ( 'NONE', *, *, #19366, .F. ) ;
#26801=EDGE_CURVE ( 'NONE', #14308, #7716, #27092, .T. ) ;
#26809=CARTESIAN_POINT ( 'NONE',  ( -104.1334669544120715, 5.043966910541457516, 5.550724164612918621 ) ) ;
#26813=CARTESIAN_POINT ( 'NONE',  ( -109.0391046861367244, -3.142556659824618404, -6.811296903636076649 ) ) ;
#26839=CARTESIAN_POINT ( 'NONE',  ( -99.91820555927569103, 0.6742432172868390028, -12.48628981526124804 ) ) ;
#26854=CARTESIAN_POINT ( 'NONE',  ( 103.4562544601546108, -5.539877390153430170, 5.057044031126181061 ) ) ;
#26856=MECHANICAL_DESIGN_GEOMETRIC_PRESENTATION_REPRESENTATION('',(#4676),#30260);
#26861=CARTESIAN_POINT ( 'NONE',  ( 129.3530333899765594, -6.000000000000000000, -57.49999999999999289 ) ) ;
#26915=DIRECTION ( 'NONE',  ( -0.000000000000000000, -0.000000000000000000, -1.000000000000000000 ) ) ;
#26965=ORIENTED_EDGE ( 'NONE', *, *, #8722, .F. ) ;
#26987=LINE ( 'NONE', #2770, #6792 ) ;
#26994=CARTESIAN_POINT ( 'NONE',  ( -109.9311937893276365, -1.369675690685145719, -7.375755714855094958 ) ) ;
#26997=ORIENTED_EDGE ( 'NONE', *, *, #11621, .F. ) ;
#27011=CARTESIAN_POINT ( 'NONE',  ( 110.7380848894539866, -2.712459438615764475E-14, -7.500000000000241585 ) ) ;
#27035=CARTESIAN_POINT ( 'NONE',  ( 110.4176386092808571, -1.928835813323004800, 7.257044673176061167 ) ) ;
#27042=EDGE_LOOP ( 'NONE', ( #8579, #28343, #2033, #23344 ) ) ;
#27092=B_SPLINE_CURVE_WITH_KNOTS ( 'NONE', 3,
 ( #26401, #9854, #13243, #29256, #23559, #17897, #4851, #26750, #7171, #12898, #28900, #10032, #15216, #18592, #20890, #7519, #28727, #18072, #34953, #21423, #4496, #2362, #29067, #26221, #15559, #31735, #10569, #31566, #10208, #20722, #7344, #23384, #4665, #12721, #21061, #18237, #29431, #32086, #7001, #7705, #26056, #2021 ),
 .UNSPECIFIED., .F., .F.,
 ( 4, 2, 2, 2, 2, 2, 2, 2, 2, 2, 2, 2, 2, 2, 2, 2, 2, 2, 2, 2, 4 ),
 ( 6.768890431529877174E-19, 0.001137415812192693870, 0.002274831624385387305, 0.003412247436578080741, 0.003980955342674426592, 0.004549663248770772876, 0.005687079060963435954, 0.006824494873156099033, 0.007393202779252448786, 0.007961910685348797673, 0.009099326497541459016, 0.009668034403637809637, 0.01023674230973416026, 0.01137415812192686150, 0.01251157393411956274, 0.01364898974631226572, 0.01478640555850496696, 0.01535511346460131411, 0.01592382137069766473, 0.01706123718289036251, 0.01819865299508306028 ),
 .UNSPECIFIED. ) ;
#27095=DIRECTION ( 'NONE',  ( -0.000000000000000000, -0.000000000000000000, -1.000000000000000000 ) ) ;
#27121=EDGE_CURVE ( 'NONE', #731, #3983, #28344, .T. ) ;
#27123=CARTESIAN_POINT ( 'NONE',  ( 129.3530333899765594, -6.000000000000000000, -62.49999999999999289 ) ) ;
#27126=CARTESIAN_POINT ( 'NONE',  ( 99.26191511054631178, -0.3844778738587134037, -12.49999999999999822 ) ) ;
#27140=VERTEX_POINT ( 'NONE', #7301 ) ;
#27153=CARTESIAN_POINT ( 'NONE',  ( -99.92067881447050581, 0.6938560566811392549, 7.475525031754233218 ) ) ;
#27205=DIRECTION ( 'NONE',  ( -0.000000000000000000, -0.000000000000000000, 1.000000000000000000 ) ) ;
#27206=CARTESIAN_POINT ( 'NONE',  ( -101.8712807483899354, -4.059672565113375597, 6.310142985817157602 ) ) ;
#27233=CARTESIAN_POINT ( 'NONE',  ( 129.3530333899765594, 6.000000000000000000, -57.49999999999999289 ) ) ;
#27292=DIRECTION ( 'NONE',  ( -0.000000000000000000, -0.000000000000000000, -1.000000000000000000 ) ) ;
#27325=CARTESIAN_POINT ( 'NONE',  ( -110.0788626153423451, 0.6978363313042807992, 7.475210363867073937 ) ) ;
#27361=EDGE_CURVE ( 'NONE', #31492, #18500, #28133, .T. ) ;
#27377=CARTESIAN_POINT ( 'NONE',  ( -104.6476413610425169, -5.105803102660849468, 5.493756281618517257 ) ) ;
#27394=ORIENTED_EDGE ( 'NONE', *, *, #4299, .F. ) ;
#27411=DIRECTION ( 'NONE',  ( 0.000000000000000000, 0.000000000000000000, 1.000000000000000000 ) ) ;
#27461=( NAMED_UNIT ( * ) SI_UNIT ( $, .STERADIAN. ) SOLID_ANGLE_UNIT ( ) );
#27467=ORIENTED_EDGE ( 'NONE', *, *, #28121, .T. ) ;
#27479=CARTESIAN_POINT ( 'NONE',  ( 100.6811048285187269, -3.796349414716898796, -11.91283353888524843 ) ) ;
#27537=CARTESIAN_POINT ( 'NONE',  ( -107.2815281471303450, 4.590414103366523335, 11.62745871345765991 ) ) ;
#27555=CARTESIAN_POINT ( 'NONE',  ( -109.4057322091481694, -2.603972021169313145, 7.035140931575562639 ) ) ;
#27558=ORIENTED_EDGE ( 'NONE', *, *, #8881, .T. ) ;
#27572=AXIS2_PLACEMENT_3D ( 'NONE', #28200, #22697, #25700 ) ;
#27615=DIRECTION ( 'NONE',  ( -0.000000000000000000, -0.000000000000000000, -1.000000000000000000 ) ) ;
#27622=ADVANCED_FACE ( 'NONE', ( #20634 ), #10123, .F. ) ;
#27654=CARTESIAN_POINT ( 'NONE',  ( 110.4388056112352956, -1.867505626284029940, -12.36477516193776260 ) ) ;
#27716=EDGE_CURVE ( 'NONE', #33784, #27140, #15659, .T. ) ;
#27717=EDGE_CURVE ( 'NONE', #109, #12045, #31307, .T. ) ;
#27723=ORIENTED_EDGE ( 'NONE', *, *, #31577, .F. ) ;
#27732=CARTESIAN_POINT ( 'NONE',  ( -109.9401885228446645, -1.370240552585045180, 7.381692049079063622 ) ) ;
#27769=EDGE_LOOP ( 'NONE', ( #4377, #10270, #6092, #10367 ) ) ;
#27778=CARTESIAN_POINT ( 'NONE',  ( -101.6217835190355885, -3.855135278743967220, -11.89320834461815934 ) ) ;
#27799=UNCERTAINTY_MEASURE_WITH_UNIT (LENGTH_MEASURE( 1.000000000000000082E-05 ), #1843, 'distance_accuracy_value', 'NONE');
#27813=DIRECTION ( 'NONE',  ( -1.000000000000000000, -0.000000000000000000, -0.000000000000000000 ) ) ;
#27826=DIRECTION ( 'NONE',  ( 0.000000000000000000, 0.000000000000000000, -1.000000000000000000 ) ) ;
#27828=CARTESIAN_POINT ( 'NONE',  ( 104.2470790493104147, -5.691643476845046123, -11.12904465084466388 ) ) ;
#27841=CARTESIAN_POINT ( 'NONE',  ( 100.0629074363043003, 2.947297676519624599, -6.904853577595275738 ) ) ;
#27847=FACE_OUTER_BOUND ( 'NONE', #27042, .T. ) ;
#27850=EDGE_CURVE ( 'NONE', #10220, #32910, #13501, .T. ) ;
#27884=LINE ( 'NONE', #5805, #19532 ) ;
#27888=AXIS2_PLACEMENT_3D ( 'NONE', #20605, #23282, #21127 ) ;
#27903=CARTESIAN_POINT ( 'NONE',  ( 105.0000000000000000, 0.000000000000000000, 57.49999999999999289 ) ) ;
#27919=EDGE_LOOP ( 'NONE', ( #20181, #636, #31769, #34503 ) ) ;
#27925=EDGE_LOOP ( 'NONE', ( #2789, #10349 ) ) ;
#27930=CARTESIAN_POINT ( 'NONE',  ( 127.4999999999999147, 0.000000000000000000, 12.50000000000000000 ) ) ;
#27937=CARTESIAN_POINT ( 'NONE',  ( -106.6595803520255430, -4.849832969747407851, 11.52164913186504869 ) ) ;
#27947=DIRECTION ( 'NONE',  ( 1.000000000000000000, 0.000000000000000000, 0.000000000000000000 ) ) ;
#27954=CARTESIAN_POINT ( 'NONE',  ( -100.3444248244574908, -2.125365432952321054, -12.31898464336051191 ) ) ;
#27978=CARTESIAN_POINT ( 'NONE',  ( -262.5000000000000000, 0.000000000000000000, 0.000000000000000000 ) ) ;
#27993=EDGE_CURVE ( 'NONE', #22922, #2593, #15672, .T. ) ;
#28067=CARTESIAN_POINT ( 'NONE',  ( -102.7226881718362392, 4.592153980832016202, 11.62674774045203385 ) ) ;
#28084=CARTESIAN_POINT ( 'NONE',  ( -99.88497961182919482, -2.585407550593147656E-15, 7.500000000000000000 ) ) ;
#28092=CARTESIAN_POINT ( 'NONE',  ( -117.4999999999997442, 0.000000000000000000, 0.000000000000000000 ) ) ;
#28104=CARTESIAN_POINT ( 'NONE',  ( 108.7927201099689682, 4.321688686550378300, 11.73238900788529726 ) ) ;
#28109=VECTOR ( 'NONE', #17330, 1000.000000000000000 ) ;
#28116=CARTESIAN_POINT ( 'NONE',  ( -102.7238790343726009, -4.592825538643425354, 11.62648616087115805 ) ) ;
#28121=EDGE_CURVE ( 'NONE', #33855, #23099, #17743, .T. ) ;
#28122=AXIS2_PLACEMENT_3D ( 'NONE', #25673, #34211, #22839 ) ;
#28133=CIRCLE ( 'NONE', #16211, 7.500000000000000000 ) ;
#28137=CARTESIAN_POINT ( 'NONE',  ( -107.5740425955733741, -4.432593925698495418, -11.68934397677214498 ) ) ;
#28170=ADVANCED_FACE ( 'NONE', ( #13632 ), #21469, .T. ) ;
#28191=PLANE ( 'NONE',  #30760 ) ;
#28194=DIRECTION ( 'NONE',  ( -1.000000000000000000, 0.000000000000000000, 0.000000000000000000 ) ) ;
#28200=CARTESIAN_POINT ( 'NONE',  ( 127.4999999999999147, 0.000000000000000000, 0.000000000000000000 ) ) ;
#28207=CARTESIAN_POINT ( 'NONE',  ( -117.4999999999997442, 0.000000000000000000, 0.000000000000000000 ) ) ;
#28218=CARTESIAN_POINT ( 'NONE',  ( 101.5039560588549676, -4.564063043377788453, -5.956988494001920209 ) ) ;
#28244=DIRECTION ( 'NONE',  ( -0.000000000000000000, -0.000000000000000000, -1.000000000000000000 ) ) ;
#28249=CARTESIAN_POINT ( 'NONE',  ( -99.91893143628131213, 0.6776097359754149618, 12.48599830169775693 ) ) ;
#28287=CARTESIAN_POINT ( 'NONE',  ( 106.5040302774077361, 5.540701522433002957, 11.20510851329258983 ) ) ;
#28300=CARTESIAN_POINT ( 'NONE',  ( -110.0732068518744597, -0.6743631657302426863, 12.48293875069316350 ) ) ;
#28317=CARTESIAN_POINT ( 'NONE',  ( -108.1252680363369336, -4.062792622693889300, -11.82295934283893146 ) ) ;
#28339=DIRECTION ( 'NONE',  ( -0.000000000000000000, -0.000000000000000000, -1.000000000000000000 ) ) ;
#28343=ORIENTED_EDGE ( 'NONE', *, *, #8888, .F. ) ;
#28344=LINE ( 'NONE', #28512, #28109 ) ;
#28374=AXIS2_PLACEMENT_3D ( 'NONE', #12651, #34348, #29004 ) ;
#28396=CARTESIAN_POINT ( 'NONE',  ( 104.2144883318369040, -5.687452395779748038, -4.889156772952023999 ) ) ;
#28454=CARTESIAN_POINT ( 'NONE',  ( 102.1101915285661050, 4.971174042719112229, 11.47116230092015421 ) ) ;
#28469=CARTESIAN_POINT ( 'NONE',  ( -130.6469666100234406, 6.000000000000000000, -62.49999999999999289 ) ) ;
#28499=EDGE_CURVE ( 'NONE', #3983, #33784, #15890, .T. ) ;
#28512=CARTESIAN_POINT ( 'NONE',  ( 129.3530333899765594, 6.000000000000000000, -57.49999999999999289 ) ) ;
#28566=AXIS2_PLACEMENT_3D ( 'NONE', #26579, #2200, #13073 ) ;
#28595=VECTOR ( 'NONE', #9297, 1000.000000000000000 ) ;
#28600=CARTESIAN_POINT ( 'NONE',  ( -109.6568079071416406, 2.122570655097208991, 12.31945284403700036 ) ) ;
#28609=CARTESIAN_POINT ( 'NONE',  ( 103.1320501907914888, -5.438347208236144148, 11.25609171608219938 ) ) ;
#28628=CARTESIAN_POINT ( 'NONE',  ( 109.3087324328219978, 3.794064876973125333, 11.91123467351735954 ) ) ;
#28664=ORIENTED_EDGE ( 'NONE', *, *, #18724, .T. ) ;
#28672=CYLINDRICAL_SURFACE ( 'NONE', #4342, 5.738084889453667792 ) ;
#28713=VECTOR ( 'NONE', #12461, 1000.000000000000000 ) ;
#28723=CARTESIAN_POINT ( 'NONE',  ( -104.6542607667447982, 5.115129524682072493, -5.485020507536669143 ) ) ;
#28727=CARTESIAN_POINT ( 'NONE',  ( 103.1339222934114588, 5.429478283318185383, -11.25942253076638089 ) ) ;
#28754=VECTOR ( 'NONE', #32809, 1000.000000000000000 ) ;
#28773=ORIENTED_EDGE ( 'NONE', *, *, #273, .T. ) ;
#28828=CIRCLE ( 'NONE', #13497, 5.115020388170798959 ) ;
#28839=ORIENTED_EDGE ( 'NONE', *, *, #10853, .T. ) ;
#28849=CARTESIAN_POINT ( 'NONE',  ( -110.1150203881707910, -1.604996202923496961E-20, 7.500000000000000000 ) ) ;
#28863=DIRECTION ( 'NONE',  ( -1.000000000000000000, 0.000000000000000000, 0.000000000000000000 ) ) ;
#28880=CARTESIAN_POINT ( 'NONE',  ( 212.5000000000000000, 0.000000000000000000, 0.000000000000000000 ) ) ;
#28884=DIRECTION ( 'NONE',  ( 0.000000000000000000, 1.000000000000000000, 0.000000000000000000 ) ) ;
#28892=CARTESIAN_POINT ( 'NONE',  ( 105.0002580737914286, 5.748131698890998287, -4.817519326574049465 ) ) ;
#28900=CARTESIAN_POINT ( 'NONE',  ( 100.8156339766184146, 3.930740943550895761, -11.86668706373619209 ) ) ;
#28941=ORIENTED_EDGE ( 'NONE', *, *, #24038, .T. ) ;
#28974=CARTESIAN_POINT ( 'NONE',  ( 129.3530333899765594, -6.000000000000000000, 62.49999999999999289 ) ) ;
#29004=DIRECTION ( 'NONE',  ( 0.000000000000000000, -0.000000000000000000, 1.000000000000000000 ) ) ;
#29017=LINE ( 'NONE', #31517, #32588 ) ;
#29041=CARTESIAN_POINT ( 'NONE',  ( -117.4999999999997442, 0.000000000000000000, 0.000000000000000000 ) ) ;
#29046=AXIS2_PLACEMENT_3D ( 'NONE', #28880, #4480, #15372 ) ;
#29059=CARTESIAN_POINT ( 'NONE',  ( 108.4984947220250291, 4.562308164568303681, -5.958384794357583836 ) ) ;
#29067=CARTESIAN_POINT ( 'NONE',  ( 105.3784337476560040, 5.728791326347600688, -11.10996872791849199 ) ) ;
#29091=ORIENTED_EDGE ( 'NONE', *, *, #14831, .F. ) ;
#29116=CARTESIAN_POINT ( 'NONE',  ( -108.8519183384634061, 3.381649300054699214, 12.03636906590513078 ) ) ;
#29148=VECTOR ( 'NONE', #23935, 1000.000000000000000 ) ;
#29152=CARTESIAN_POINT ( 'NONE',  ( 99.77797576327679963, 2.385570507987203825, 12.27149918290385244 ) ) ;
#29198=B_SPLINE_CURVE_WITH_KNOTS ( 'NONE', 3,
 ( #14268, #30458, #31162, #19785, #19612, #9266, #22797, #27954, #3389, #33115, #20132, #912, #9454, #27778, #1261, #11780, #22630, #8731, #33647, #556, #33469, #17487, #19956, #6761, #22271, #30808, #28137, #28317, #6585, #733, #3908, #14800, #25627, #11411, #12130, #22971, #6050, #33826, #25098, #23320 ),
 .UNSPECIFIED., .F., .F.,
 ( 4, 2, 2, 2, 2, 2, 2, 2, 2, 2, 2, 2, 2, 2, 2, 2, 2, 2, 2, 4 ),
 ( 0.01617148595533311056, 0.01667647242675793923, 0.01718145889818276789, 0.01819143184103242522, 0.01869641831245725735, 0.01920140478388208602, 0.02021137772673176763, 0.02122135066958145272, 0.02223132361243113433, 0.02324129655528081595, 0.02425126949813049756, 0.02526124244098017918, 0.02627121538382986080, 0.02728118832667954241, 0.02829116126952922403, 0.02879614774095407698, 0.02930113421237893340, 0.03031110715522863930, 0.03132108009807835214, 0.03233105304092805804 ),
 .UNSPECIFIED. ) ;
#29218=EDGE_LOOP ( 'NONE', ( #6184, #19061, #13162, #14958 ) ) ;
#29235=CARTESIAN_POINT ( 'NONE',  ( -105.0000000000000000, 0.000000000000000000, 60.00000000000000000 ) ) ;
#29247=CARTESIAN_POINT ( 'NONE',  ( 110.1126341753765416, 2.611822472857947108, -7.032742872185955285 ) ) ;
#29256=CARTESIAN_POINT ( 'NONE',  ( 99.44953031585586700, 1.503590720865120911, -12.41481623251361555 ) ) ;
#29257=( NAMED_UNIT ( * ) SI_UNIT ( $, .STERADIAN. ) SOLID_ANGLE_UNIT ( ) );
#29315=CARTESIAN_POINT ( 'NONE',  ( 110.2199516832989730, -2.390228624448382799, 12.27061385718275943 ) ) ;
#29341=CARTESIAN_POINT ( 'NONE',  ( -107.2773118281637039, 4.592153980832013538, -11.62674774045203208 ) ) ;
#29351=AXIS2_PLACEMENT_3D ( 'NONE', #19448, #27615, #3229 ) ;
#29355=ORIENTED_EDGE ( 'NONE', *, *, #17469, .F. ) ;
#29361=CARTESIAN_POINT ( 'NONE',  ( 106.9039025905678955, -5.425683864377651489, 5.182047996533464485 ) ) ;
#29376=DIRECTION ( 'NONE',  ( 0.7071067811865512365, 8.659560562354889717E-17, 0.7071067811865439090 ) ) ;
#29420=LINE ( 'NONE', #2183, #31574 ) ;
#29428=CARTESIAN_POINT ( 'NONE',  ( -100.9340356286931097, 3.171022835462805389, -6.816853140736490957 ) ) ;
#29431=CARTESIAN_POINT ( 'NONE',  ( 110.2220242367232146, 2.385570507987203825, -12.27149918290385600 ) ) ;
#29437=EDGE_CURVE ( 'NONE', #1125, #5515, #5885, .T. ) ;
#29444=ORIENTED_EDGE ( 'NONE', *, *, #27993, .F. ) ;
#29453=ORIENTED_EDGE ( 'NONE', *, *, #7789, .T. ) ;
#29464=ORIENTED_EDGE ( 'NONE', *, *, #13875, .T. ) ;
#29495=CARTESIAN_POINT ( 'NONE',  ( -108.7214454096172460, -3.512874579320472979, -6.627714125729964323 ) ) ;
#29518=ORIENTED_EDGE ( 'NONE', *, *, #8722, .T. ) ;
#29536=CARTESIAN_POINT ( 'NONE',  ( 102.4159735622909722, -5.136475861867761061, 5.468785347707075140 ) ) ;
#29545=EDGE_CURVE ( 'NONE', #8598, #109, #31335, .T. ) ;
#29571=EDGE_LOOP ( 'NONE', ( #25777, #4693, #33209, #27723 ) ) ;
#29592=AXIS2_PLACEMENT_3D ( 'NONE', #20961, #4394, #23806 ) ;
#29593=DIRECTION ( 'NONE',  ( -1.000000000000000000, -0.000000000000000000, -0.000000000000000000 ) ) ;
#29626=DIRECTION ( 'NONE',  ( -0.000000000000000000, -0.000000000000000000, -1.000000000000000000 ) ) ;
#29628=DIRECTION ( 'NONE',  ( -0.000000000000000000, -0.000000000000000000, -1.000000000000000000 ) ) ;
#29634=DIRECTION ( 'NONE',  ( 0.000000000000000000, 0.000000000000000000, 1.000000000000000000 ) ) ;
#29645=EDGE_CURVE ( 'NONE', #22922, #32630, #5143, .T. ) ;
#29663=CARTESIAN_POINT ( 'NONE',  ( -108.8307179568225109, -3.393468573754154782, -6.689828017866635612 ) ) ;
#29675=DIRECTION ( 'NONE',  ( 0.000000000000000000, 0.000000000000000000, -1.000000000000000000 ) ) ;
#29684=CARTESIAN_POINT ( 'NONE',  ( 105.0000000000000000, 0.000000000000000000, 60.00000000000000000 ) ) ;
#29801=CARTESIAN_POINT ( 'NONE',  ( 101.2096900042061804, -4.324196401257808908, -11.73154709691606179 ) ) ;
#29835=CARTESIAN_POINT ( 'NONE',  ( -100.5859555588355079, 2.605551551359105211, 7.039079951515508249 ) ) ;
#29848=DIRECTION ( 'NONE',  ( 0.000000000000000000, 0.000000000000000000, -1.000000000000000000 ) ) ;
#29857=VECTOR ( 'NONE', #3100, 1000.000000000000000 ) ;
#29861=APPLICATION_CONTEXT ( 'automotive_design' ) ;
#29885=CARTESIAN_POINT ( 'NONE',  ( -99.92078033151290128, -0.6954373895739828226, 7.475453221064620735 ) ) ;
#29910=DIRECTION ( 'NONE',  ( 1.000000000000000000, -0.000000000000000000, -0.000000000000000000 ) ) ;
#29929=CARTESIAN_POINT ( 'NONE',  ( -262.5000000000000000, 0.000000000000000000, 7.500000000000000000 ) ) ;
#29950=DIRECTION ( 'NONE',  ( -0.000000000000000000, -0.000000000000000000, -1.000000000000000000 ) ) ;
#29978=CARTESIAN_POINT ( 'NONE',  ( 99.86204640771551055, -2.561659524636490826, -12.23586498300002035 ) ) ;
#30000=AXIS2_PLACEMENT_3D ( 'NONE', #33806, #22607, #25254 ) ;
#30014=AXIS2_PLACEMENT_3D ( 'NONE', #8429, #24431, #16285 ) ;
#30040=CARTESIAN_POINT ( 'NONE',  ( -108.8478167861455148, 3.386225727737903757, -12.03506400121763775 ) ) ;
#30047=EDGE_CURVE ( 'NONE', #9756, #30505, #12643, .T. ) ;
#30059=DIRECTION ( 'NONE',  ( 1.000000000000000000, 0.000000000000000000, 0.000000000000000000 ) ) ;
#30060=CARTESIAN_POINT ( 'NONE',  ( -107.2949071119419813, -4.583230167788450160, 5.938965658480642951 ) ) ;
#30067=CYLINDRICAL_SURFACE ( 'NONE', #1789, 12.50000000000000000 ) ;
#30095=EDGE_LOOP ( 'NONE', ( #18189, #12685, #13625, #17295 ) ) ;
#30104=VERTEX_POINT ( 'NONE', #26479 ) ;
#30144=CARTESIAN_POINT ( 'NONE',  ( 106.8679498092085538, -5.438347208236144148, -11.25609171608219938 ) ) ;
#30176=DIRECTION ( 'NONE',  ( -0.000000000000000000, -0.000000000000000000, -1.000000000000000000 ) ) ;
#30206=CARTESIAN_POINT ( 'NONE',  ( -105.6777138778371068, 5.081071289440263428, 11.42094332255972589 ) ) ;
#30224=CARTESIAN_POINT ( 'NONE',  ( -101.1692820431775033, -3.393468573754153006, 6.689828017866632948 ) ) ;
#30260=( GEOMETRIC_REPRESENTATION_CONTEXT ( 3 ) GLOBAL_UNCERTAINTY_ASSIGNED_CONTEXT ( ( #27799 ) ) GLOBAL_UNIT_ASSIGNED_CONTEXT ( ( #1843, #7345, #29257 ) ) REPRESENTATION_CONTEXT ( 'NONE', 'WORKASPACE' ) );
#30276=ORIENTED_EDGE ( 'NONE', *, *, #17469, .T. ) ;
#30301=AXIS2_PLACEMENT_3D ( 'NONE', #1149, #17189, #20025 ) ;
#30356=CARTESIAN_POINT ( 'NONE',  ( 129.3530333899765594, 6.000000000000000000, -62.49999999999999289 ) ) ;
#30370=VECTOR ( 'NONE', #5303, 1000.000000000000000 ) ;
#30386=DIRECTION ( 'NONE',  ( -0.000000000000000000, -0.000000000000000000, -1.000000000000000000 ) ) ;
#30408=CARTESIAN_POINT ( 'NONE',  ( 110.1903123430731881, -2.454113965193227997, 7.089506392665936296 ) ) ;
#30411=EDGE_LOOP ( 'NONE', ( #29444, #15473, #24501, #5007 ) ) ;
#30439=VECTOR ( 'NONE', #23212, 1000.000000000000000 ) ;
#30458=CARTESIAN_POINT ( 'NONE',  ( -99.88497961182919482, -0.1683156175999579174, -12.50000000000000000 ) ) ;
#30462=LINE ( 'NONE', #3566, #10715 ) ;
#30471=CYLINDRICAL_SURFACE ( 'NONE', #29351, 5.738084889453667792 ) ;
#30505=VERTEX_POINT ( 'NONE', #1872 ) ;
#30511=CARTESIAN_POINT ( 'NONE',  ( 109.8644316410288013, -3.049149995829645299, -12.12344935835687920 ) ) ;
#30542=CARTESIAN_POINT ( 'NONE',  ( 101.2273074351206503, -4.338569679229816067, -6.125236864567445316 ) ) ;
#30584=EDGE_LOOP ( 'NONE', ( #8289, #34204, #16053, #18425 ) ) ;
#30698=CARTESIAN_POINT ( 'NONE',  ( 99.30309277135016544, 0.7888478034546075879, -7.468363897292212172 ) ) ;
#30713=CARTESIAN_POINT ( 'NONE',  ( 100.7124613249971503, -3.830588487554197119, -6.455099174110775273 ) ) ;
#30733=ADVANCED_FACE ( 'NONE', ( #3277 ), #24106, .F. ) ;
#30741=CARTESIAN_POINT ( 'NONE',  ( -99.88497961182919482, 6.264093345946821604E-16, 12.50000000000000000 ) ) ;
#30760=AXIS2_PLACEMENT_3D ( 'NONE', #17007, #14853, #22323 ) ;
#30779=AXIS2_PLACEMENT_3D ( 'NONE', #12289, #18161, #33980 ) ;
#30788=CARTESIAN_POINT ( 'NONE',  ( -99.91951324175876437, -0.6815953102691991727, 12.48576125250277968 ) ) ;
#30808=CARTESIAN_POINT ( 'NONE',  ( -107.2761209656274417, -4.592825538643426242, -11.62648616087116160 ) ) ;
#30818=ORIENTED_EDGE ( 'NONE', *, *, #18724, .F. ) ;
#30828=CARTESIAN_POINT ( 'NONE',  ( 105.0000000000000000, 0.000000000000000000, 60.00000000000000000 ) ) ;
#30876=VECTOR ( 'NONE', #31643, 1000.000000000000000 ) ;
#30885=CARTESIAN_POINT ( 'NONE',  ( 102.4141533279665026, -5.135784989587515170, -5.469495349232144754 ) ) ;
#30943=VECTOR ( 'NONE', #10798, 1000.000000000000000 ) ;
#30953=CARTESIAN_POINT ( 'NONE',  ( 110.7380848894536882, 0.3849557905273008340, 12.50000000000000533 ) ) ;
#30964=DIRECTION ( 'NONE',  ( -0.7071067811865435759, 8.659560562354980929E-17, -0.7071067811865514585 ) ) ;
#30965=CARTESIAN_POINT ( 'NONE',  ( -100.9438390900021432, -3.120668149329707486, 12.10491939767606873 ) ) ;
#31046=ORIENTED_EDGE ( 'NONE', *, *, #6425, .F. ) ;
#31067=CARTESIAN_POINT ( 'NONE',  ( 108.4931367044692934, -4.566352457759228045, -5.955250171528614800 ) ) ;
#31115=DIRECTION ( 'NONE',  ( 1.000000000000000000, 0.000000000000000000, 0.000000000000000000 ) ) ;
#31133=CARTESIAN_POINT ( 'NONE',  ( 103.1340045722813130, 5.439315735761663717, 11.25565174199232743 ) ) ;
#31146=CARTESIAN_POINT ( 'NONE',  ( -110.1150203881708336, -0.1683156175999609427, 12.50000000000000000 ) ) ;
#31150=VERTEX_POINT ( 'NONE', #14247 ) ;
#31162=CARTESIAN_POINT ( 'NONE',  ( -99.89326661827516318, -0.3368495349214569723, -12.49660185505138976 ) ) ;
#31180=EDGE_CURVE ( 'NONE', #19820, #9756, #17097, .T. ) ;
#31190=CIRCLE ( 'NONE', #6736, 10.00000000000000000 ) ;
#31204=ORIENTED_EDGE ( 'NONE', *, *, #23148, .F. ) ;
#31216=CARTESIAN_POINT ( 'NONE',  ( 129.3530333899765594, 6.000000000000000000, 62.49999999999999289 ) ) ;
#31237=CARTESIAN_POINT ( 'NONE',  ( 107.5840264377090421, -5.136475861867761061, -5.468785347707075140 ) ) ;
#31269=ADVANCED_FACE ( 'NONE', ( #22774 ), #11931, .T. ) ;
#31278=CARTESIAN_POINT ( 'NONE',  ( 99.26191511054632599, 1.643815732525060864E-21, 12.50000000000000000 ) ) ;
#31294=CARTESIAN_POINT ( 'NONE',  ( 100.6806599292393116, 3.795444455902926340, 11.91305592319908691 ) ) ;
#31306=UNCERTAINTY_MEASURE_WITH_UNIT (LENGTH_MEASURE( 1.000000000000000082E-05 ), #16628, 'distance_accuracy_value', 'NONE');
#31307=LINE ( 'NONE', #20462, #28713 ) ;
#31314=EDGE_CURVE ( 'NONE', #13351, #33784, #1748, .T. ) ;
#31331=AXIS2_PLACEMENT_3D ( 'NONE', #17987, #9948, #34330 ) ;
#31335=LINE ( 'NONE', #25465, #18843 ) ;
#31347=CARTESIAN_POINT ( 'NONE',  ( -117.4999999999997442, 0.000000000000000000, 12.50000000000000000 ) ) ;
#31367=ADVANCED_FACE ( 'NONE', ( #13148 ), #2269, .T. ) ;
#31393=CARTESIAN_POINT ( 'NONE',  ( -105.3514761500790655, 5.105882603317796864, -5.493682664683364081 ) ) ;
#31395=EDGE_LOOP ( 'NONE', ( #8273, #29091, #24089, #2735 ) ) ;
#31404=VECTOR ( 'NONE', #33804, 1000.000000000000000 ) ;
#31469=EDGE_CURVE ( 'NONE', #7139, #20721, #9943, .T. ) ;
#31490=CARTESIAN_POINT ( 'NONE',  ( 109.2875386750028639, -3.830588487554197119, 6.455099174110775273 ) ) ;
#31492=VERTEX_POINT ( 'NONE', #16883 ) ;
#31503=EDGE_CURVE ( 'NONE', #30505, #8267, #27884, .T. ) ;
#31517=CARTESIAN_POINT ( 'NONE',  ( 127.4999999999999147, 0.000000000000000000, 2.499999999999825473 ) ) ;
#31536=CARTESIAN_POINT ( 'NONE',  ( -130.6469666100234406, 6.000000000000000000, -62.49999999999999289 ) ) ;
#31540=FACE_OUTER_BOUND ( 'NONE', #30411, .T. ) ;
#31561=CARTESIAN_POINT ( 'NONE',  ( 104.6072996318409736, 5.728044018051756225, -4.841538128164400767 ) ) ;
#31563=CARTESIAN_POINT ( 'NONE',  ( -107.5866028038673932, 4.424631548980197948, -6.059743929710635690 ) ) ;
#31566=CARTESIAN_POINT ( 'NONE',  ( 107.5624465017048550, 5.148005685260259590, -11.39183432441182653 ) ) ;
#31574=VECTOR ( 'NONE', #28884, 1000.000000000000000 ) ;
#31577=EDGE_CURVE ( 'NONE', #2811, #6643, #187, .T. ) ;
#31591=CARTESIAN_POINT ( 'NONE',  ( -105.0000000000000000, 0.000000000000000000, -57.49999999999999289 ) ) ;
#31621=CARTESIAN_POINT ( 'NONE',  ( 106.5040163601712351, -5.550599894338584583, 11.20035359757823912 ) ) ;
#31626=CARTESIAN_POINT ( 'NONE',  ( -103.3138017543800373, -4.840385614786930191, -5.731315639859864142 ) ) ;
#31643=DIRECTION ( 'NONE',  ( -1.000000000000000000, -0.000000000000000000, -0.000000000000000000 ) ) ;
#31663=CARTESIAN_POINT ( 'NONE',  ( 99.31309745116723775, -0.7897130297925551989, 7.460902677354920520 ) ) ;
#31729=CARTESIAN_POINT ( 'NONE',  ( 107.0789465421990201, 5.351410369513340370, -5.255735268165820706 ) ) ;
#31735=CARTESIAN_POINT ( 'NONE',  ( 106.5032006809128546, 5.550581019792740989, -11.20035861729703797 ) ) ;
#31741=LINE ( 'NONE', #33585, #1278 ) ;
#31769=ORIENTED_EDGE ( 'NONE', *, *, #8635, .F. ) ;
#31844=CARTESIAN_POINT ( 'NONE',  ( -117.4999999999997442, 1.530808498934191521E-15, 12.50000000000000000 ) ) ;
#31866=CARTESIAN_POINT ( 'NONE',  ( 107.0769369097902057, 5.352195967840122748, 5.254935570228769670 ) ) ;
#31870=AXIS2_PLACEMENT_3D ( 'NONE', #24990, #19680, #3456 ) ;
#31898=CARTESIAN_POINT ( 'NONE',  ( -109.8372293046274137, 1.696271239234544037, -7.312686146626635519 ) ) ;
#31931=CARTESIAN_POINT ( 'NONE',  ( 129.3530333899765594, 6.000000000000000000, -62.49999999999999289 ) ) ;
#31943=ORIENTED_EDGE ( 'NONE', *, *, #29437, .T. ) ;
#31981=AXIS2_PLACEMENT_3D ( 'NONE', #29684, #15471, #7961 ) ;
#31989=CARTESIAN_POINT ( 'NONE',  ( 99.56190681375883855, 1.868749050043680082, 12.36447865323539652 ) ) ;
#31994=CARTESIAN_POINT ( 'NONE',  ( -109.5901181662249542, 2.281765576240578852, -12.29396198687796726 ) ) ;
#32033=ORIENTED_EDGE ( 'NONE', *, *, #18867, .F. ) ;
#32078=CARTESIAN_POINT ( 'NONE',  ( 105.9796427714311733, 5.657131480001861057, -4.924467467246998353 ) ) ;
#32086=CARTESIAN_POINT ( 'NONE',  ( 110.4380931862411899, 1.868749050043681192, -12.36447865323539475 ) ) ;
#32095=ORIENTED_EDGE ( 'NONE', *, *, #23297, .F. ) ;
#32154=CARTESIAN_POINT ( 'NONE',  ( -108.1287192516100504, -4.059672565113384479, -6.310142985817148720 ) ) ;
#32155=FACE_OUTER_BOUND ( 'NONE', #27769, .T. ) ;
#32197=FACE_OUTER_BOUND ( 'NONE', #10145, .T. ) ;
#32198=CARTESIAN_POINT ( 'NONE',  ( 129.3530333899765594, 6.000000000000000000, 62.49999999999999289 ) ) ;
#32237=CARTESIAN_POINT ( 'NONE',  ( 106.9002205115570376, 5.417593104495392886, 5.187149597110491506 ) ) ;
#32260=CARTESIAN_POINT ( 'NONE',  ( -99.88497961182919482, 6.264093345946821604E-16, 60.00000000000000000 ) ) ;
#32282=ORIENTED_EDGE ( 'NONE', *, *, #3704, .F. ) ;
#32296=DIRECTION ( 'NONE',  ( -1.000000000000000000, -0.000000000000000000, -0.000000000000000000 ) ) ;
#32316=CARTESIAN_POINT ( 'NONE',  ( -103.3063056233373089, 4.837773223901916886, 5.733537676439135033 ) ) ;
#32318=CARTESIAN_POINT ( 'NONE',  ( -0.000000000000000000, 0.000000000000000000, 57.49999999999999289 ) ) ;
#32321=CARTESIAN_POINT ( 'NONE',  ( -99.88497961182920903, -0.1727115935459978269, -7.500000000000000888 ) ) ;
#32334=DIRECTION ( 'NONE',  ( 0.000000000000000000, 0.000000000000000000, 1.000000000000000000 ) ) ;
#32347=CARTESIAN_POINT ( 'NONE',  ( -99.88497961182919482, 0.3368795255050330839, -12.50000000000000178 ) ) ;
#32365=CARTESIAN_POINT ( 'NONE',  ( 110.7380848894536598, -0.3983872338823410408, 7.499999999999998224 ) ) ;
#32369=CARTESIAN_POINT ( 'NONE',  ( -99.88497961182919482, 6.264093345946822590E-16, 57.49999999999999289 ) ) ;
#32434=CARTESIAN_POINT ( 'NONE',  ( 110.7277013283863170, -0.3974226492620277496, -7.492047161373153408 ) ) ;
#32456=CARTESIAN_POINT ( 'NONE',  ( 105.9525633024387332, -5.661646449284257976, -11.14439484353662735 ) ) ;
#32489=ORIENTED_EDGE ( 'NONE', *, *, #10253, .F. ) ;
#32506=DIRECTION ( 'NONE',  ( 0.000000000000000000, -1.000000000000000000, -0.000000000000000000 ) ) ;
#32533=( GEOMETRIC_REPRESENTATION_CONTEXT ( 3 ) GLOBAL_UNCERTAINTY_ASSIGNED_CONTEXT ( ( #31306 ) ) GLOBAL_UNIT_ASSIGNED_CONTEXT ( ( #16628, #17336, #27461 ) ) REPRESENTATION_CONTEXT ( 'NONE', 'WORKASPACE' ) );
#32536=CARTESIAN_POINT ( 'NONE',  ( -108.8320610496387246, -3.403480489512942686, 6.688370467007148434 ) ) ;
#32577=CARTESIAN_POINT ( 'NONE',  ( 99.65514493969531884, 2.096151729099205774, 7.203423290846323823 ) ) ;
#32588=VECTOR ( 'NONE', #15507, 1000.000000000000000 ) ;
#32630=VERTEX_POINT ( 'NONE', #31347 ) ;
#32633=CARTESIAN_POINT ( 'NONE',  ( 99.78004831670104124, -2.390228624448383243, -12.27061385718275943 ) ) ;
#32661=DIRECTION ( 'NONE',  ( 0.000000000000000000, 1.000000000000000000, 0.000000000000000000 ) ) ;
#32670=CARTESIAN_POINT ( 'NONE',  ( -107.7224926025144498, 4.333302303957496271, 6.122453330911801217 ) ) ;
#32702=CARTESIAN_POINT ( 'NONE',  ( -106.8169753891507838, 4.784316299155410235, -11.54838096230724176 ) ) ;
#32719=CARTESIAN_POINT ( 'NONE',  ( -110.1150203881707910, -0.1727115935459996587, 7.500000000000000888 ) ) ;
#32748=DIRECTION ( 'NONE',  ( -1.000000000000000000, 0.000000000000000000, 0.000000000000000000 ) ) ;
#32771=DIRECTION ( 'NONE',  ( -1.000000000000000000, 0.000000000000000000, 0.000000000000000000 ) ) ;
#32776=CARTESIAN_POINT ( 'NONE',  ( 110.7380848894536598, 7.027143731242819742E-16, -12.50000000000000000 ) ) ;
#32784=CARTESIAN_POINT ( 'NONE',  ( -99.88497961182923746, 0.3459610470522913594, -7.500000000000001776 ) ) ;
#32792=CARTESIAN_POINT ( 'NONE',  ( 110.5373916640127590, -1.553728400065965687, -7.347407880389961399 ) ) ;
#32797=ORIENTED_EDGE ( 'NONE', *, *, #22356, .T. ) ;
#32809=DIRECTION ( 'NONE',  ( -1.000000000000000000, -0.000000000000000000, -0.000000000000000000 ) ) ;
#32811=CARTESIAN_POINT ( 'NONE',  ( 110.1383142917281646, -2.560920621327495983, -12.23601723495363380 ) ) ;
#32832=ORIENTED_EDGE ( 'NONE', *, *, #35084, .T. ) ;
#32837=AXIS2_PLACEMENT_3D ( 'NONE', #21968, #24616, #27826 ) ;
#32840=CARTESIAN_POINT ( 'NONE',  ( -110.1150203881707625, 0.3459610470522903047, 7.499999999999997335 ) ) ;
#32874=CARTESIAN_POINT ( 'NONE',  ( -104.6588445208797822, 5.114806216612618250, 11.40564585725303992 ) ) ;
#32893=CARTESIAN_POINT ( 'NONE',  ( 110.7380848894536598, -4.118294838564020743E-16, 7.500000000000000000 ) ) ;
#32910=VERTEX_POINT ( 'NONE', #9333 ) ;
#32932=CARTESIAN_POINT ( 'NONE',  ( 99.80463941335877109, 2.443267496989373733, 7.093208238637026319 ) ) ;
#32980=CARTESIAN_POINT ( 'NONE',  ( 105.7618603918998303, -5.690476701307018104, -11.12964202013672654 ) ) ;
#32986=DIRECTION ( 'NONE',  ( -0.000000000000000000, -0.000000000000000000, -1.000000000000000000 ) ) ;
#33008=DIRECTION ( 'NONE',  ( -0.000000000000000000, 0.000000000000000000, -1.000000000000000000 ) ) ;
#33027=DIRECTION ( 'NONE',  ( -1.000000000000000000, 0.000000000000000000, 0.000000000000000000 ) ) ;
#33040=CARTESIAN_POINT ( 'NONE',  ( 105.0000000000000000, 0.000000000000000000, -57.49999999999999289 ) ) ;
#33048=ORIENTED_EDGE ( 'NONE', *, *, #18123, .F. ) ;
#33063=CARTESIAN_POINT ( 'NONE',  ( -99.88497961182919482, -2.585407550593147656E-15, 7.500000000000000000 ) ) ;
#33096=CARTESIAN_POINT ( 'NONE',  ( -108.3782164809644115, -3.855135278743967664, 11.89320834461816112 ) ) ;
#33108=B_SPLINE_CURVE_WITH_KNOTS ( 'NONE', 3,
 ( #31278, #20600, #7055, #4546, #15623, #34294, #12596, #4209, #17769, #7398, #34473, #4381, #15095, #20432, #25939, #15271, #1894, #28609, #12951, #26109, #1723, #23439, #9913, #20774, #1556, #23793, #31621, #18476, #33950, #15442, #26281, #21118, #18295, #12430, #12777, #23619, #10089, #29315, #4905, #15802, #23277, #23105, #26633 ),
 .UNSPECIFIED., .F., .F.,
 ( 4, 2, 2, 2, 2, 2, 2, 2, 2, 2, 2, 1, 2, 2, 2, 2, 2, 2, 2, 2, 2, 4 ),
 ( 0.01819865299508306375, 0.01933465672311147215, 0.02047066045113988403, 0.02103866231515407956, 0.02160666417916827509, 0.02217466604318247062, 0.02274266790719666614, 0.02387867163522502945, 0.02501467536325339275, 0.02615067909128175605, 0.02671868095529594117, 0.02728668281931011935, 0.02785468468332430100, 0.02842268654733848265, 0.02955869027536688412, 0.03069469400339528906, 0.03183069773142369052, 0.03296670145945209546, 0.03353470332346629446, 0.03410270518748049345, 0.03523870891550889839, 0.03637471264353730332 ),
 .UNSPECIFIED. ) ;
#33115=CARTESIAN_POINT ( 'NONE',  ( -100.5759650167679951, -2.572809509134356354, -12.23328267615805665 ) ) ;
#33118=DIRECTION ( 'NONE',  ( 1.000000000000000000, -0.000000000000000000, -0.000000000000000000 ) ) ;
#33154=B_SPLINE_CURVE_WITH_KNOTS ( 'NONE', 3,
 ( #27011, #21596, #32434, #16447, #8058, #32792, #18936, #8416, #19289, #6834, #19871, #12385, #31067, #22884, #31237, #14713, #11862, #3985, #14882, #25535, #3640, #17390, #811, #28396, #3818, #15055, #8815, #30885, #9530, #28218, #30542, #30713, #23232, #12215, #17727, #33549, #33729, #1344, #1164, #12036, #1513, #19691 ),
 .UNSPECIFIED., .F., .F.,
 ( 4, 2, 2, 2, 2, 2, 2, 2, 2, 2, 2, 2, 2, 2, 2, 2, 2, 2, 2, 2, 4 ),
 ( 0.01884718663114543988, 0.01943499450852638824, 0.02002280238590734007, 0.02119841814066924027, 0.02237403389543114046, 0.02354964965019304066, 0.02472526540495494085, 0.02590088115971684452, 0.02707649691447874471, 0.02766430479185969654, 0.02825211266924064490, 0.02883992054662159674, 0.02942772842400254510, 0.03060334417876444529, 0.03177895993352634896, 0.03295457568828825262, 0.03413019144305015629, 0.03471799932043109771, 0.03530580719781203913, 0.03648142295257392198, 0.03765703870733580483 ),
 .UNSPECIFIED. ) ;
#33179=PRODUCT_DEFINITION_FORMATION_WITH_SPECIFIED_SOURCE ( 'ANY', '', #22286, .NOT_KNOWN. ) ;
#33188=CARTESIAN_POINT ( 'NONE',  ( 110.7380848894536598, 7.027127293105237708E-16, 57.49999999999999289 ) ) ;
#33209=ORIENTED_EDGE ( 'NONE', *, *, #18858, .T. ) ;
#33372=ORIENTED_EDGE ( 'NONE', *, *, #273, .F. ) ;
#33454=CARTESIAN_POINT ( 'NONE',  ( -109.4240349832319907, -2.572809509134357242, 12.23328267615805132 ) ) ;
#33469=CARTESIAN_POINT ( 'NONE',  ( -104.6618752167676973, -5.114954807106460777, -11.40557921924218832 ) ) ;
#33492=CYLINDRICAL_SURFACE ( 'NONE', #21933, 5.738084889453667792 ) ;
#33533=CARTESIAN_POINT ( 'NONE',  ( 101.2248971821314569, 4.336304859840375059, -6.126759150192703451 ) ) ;
#33542=EDGE_LOOP ( 'NONE', ( #11235, #28773, #20897, #32282 ) ) ;
#33549=CARTESIAN_POINT ( 'NONE',  ( 99.89373959579265261, -2.624171310066655938, -7.028111897042786715 ) ) ;
#33585=CARTESIAN_POINT ( 'NONE',  ( -110.1150203881707910, 0.000000000000000000, 60.00000000000000000 ) ) ;
#33597=CARTESIAN_POINT ( 'NONE',  ( -110.1150203881707910, 0.000000000000000000, -57.49999999999999289 ) ) ;
#33618=AXIS2_PLACEMENT_3D ( 'NONE', #20843, #9987, #2152 ) ;
#33627=LINE ( 'NONE', #17101, #17286 ) ;
#33629=CARTESIAN_POINT ( 'NONE',  ( -109.3380992783527432, -2.715097909449874614, 12.20238416997438158 ) ) ;
#33647=CARTESIAN_POINT ( 'NONE',  ( -103.6592623599142087, -4.947629808455840994, -11.47938275244241169 ) ) ;
#33651=ORIENTED_EDGE ( 'NONE', *, *, #435, .F. ) ;
#33712=CYLINDRICAL_SURFACE ( 'NONE', #27572, 12.50000000000000000 ) ;
#33729=CARTESIAN_POINT ( 'NONE',  ( 99.80968765692681188, -2.454113965193227997, -7.089506392665936296 ) ) ;
#33765=CIRCLE ( 'NONE', #17326, 7.500000000000000000 ) ;
#33784=VERTEX_POINT ( 'NONE', #21801 ) ;
#33786=ORIENTED_EDGE ( 'NONE', *, *, #7135, .T. ) ;
#33804=DIRECTION ( 'NONE',  ( -1.000000000000000000, -0.000000000000000000, -0.000000000000000000 ) ) ;
#33806=CARTESIAN_POINT ( 'NONE',  ( -105.0000000000000000, 0.000000000000000000, 60.00000000000000000 ) ) ;
#33807=CARTESIAN_POINT ( 'NONE',  ( -99.88497961182919482, 9.184690493976639608E-16, -7.500000000000000000 ) ) ;
#33811=LINE ( 'NONE', #20635, #21142 ) ;
#33819=VECTOR ( 'NONE', #25407, 1000.000000000000000 ) ;
#33826=CARTESIAN_POINT ( 'NONE',  ( -110.0804867582412214, -0.6815953102692046128, -12.48576125250277968 ) ) ;
#33831=CARTESIAN_POINT ( 'NONE',  ( 212.5000000000000000, 0.000000000000000000, 7.500000000000000000 ) ) ;
#33839=VECTOR ( 'NONE', #25495, 1000.000000000000000 ) ;
#33843=EDGE_LOOP ( 'NONE', ( #8767, #8570 ) ) ;
#33855=VERTEX_POINT ( 'NONE', #33188 ) ;
#33879=EDGE_CURVE ( 'NONE', #24651, #6202, #12020, .T. ) ;
#33938=CARTESIAN_POINT ( 'NONE',  ( -108.3843351873371574, 3.849558703864948583, 11.89498339909459723 ) ) ;
#33950=CARTESIAN_POINT ( 'NONE',  ( 107.5556592954127666, -5.151199242560473124, 11.39037137834242586 ) ) ;
#33972=CARTESIAN_POINT ( 'NONE',  ( 107.0424307436086337, 5.365524250098477665, 11.29014866489560376 ) ) ;
#33980=DIRECTION ( 'NONE',  ( 0.000000000000000000, 0.000000000000000000, 1.000000000000000000 ) ) ;
#33982=CARTESIAN_POINT ( 'NONE',  ( -130.6469666100234406, 6.000000000000000000, -57.49999999999999289 ) ) ;
#34050=CARTESIAN_POINT ( 'NONE',  ( 119.9999999999998295, 0.000000000000000000, 10.00000000000000000 ) ) ;
#34055=MANIFOLD_SOLID_BREP ( 'Boss-Extrude5', #10361 ) ;
#34071=VERTEX_POINT ( 'NONE', #19119 ) ;
#34105=CARTESIAN_POINT ( 'NONE',  ( -110.1150203881707910, 3.166944581793445397E-20, 12.50000000000000000 ) ) ;
#34123=EDGE_LOOP ( 'NONE', ( #25674, #3602, #21581, #25107 ) ) ;
#34170=VECTOR ( 'NONE', #29376, 1000.000000000000000 ) ;
#34204=ORIENTED_EDGE ( 'NONE', *, *, #4110, .F. ) ;
#34211=DIRECTION ( 'NONE',  ( -1.000000000000000000, -0.000000000000000000, -0.000000000000000000 ) ) ;
#34216=ORIENTED_EDGE ( 'NONE', *, *, #26801, .T. ) ;
#34250=VECTOR ( 'NONE', #12455, 1000.000000000000000 ) ;
#34285=CARTESIAN_POINT ( 'NONE',  ( -108.1244492803746766, 4.063381404898920302, 11.82275161328742286 ) ) ;
#34294=CARTESIAN_POINT ( 'NONE',  ( 99.77990078431651000, -2.389942209051219901, 12.27067588826158762 ) ) ;
#34317=CARTESIAN_POINT ( 'NONE',  ( 100.0353719831124977, 2.883232572601701627, 12.16410353805738964 ) ) ;
#34330=DIRECTION ( 'NONE',  ( 0.000000000000000000, 0.000000000000000000, 1.000000000000000000 ) ) ;
#34341=CARTESIAN_POINT ( 'NONE',  ( 99.34337556290111593, -0.9828571727418841109, 7.437816238889399578 ) ) ;
#34348=DIRECTION ( 'NONE',  ( 0.000000000000000000, 1.000000000000000000, 0.000000000000000000 ) ) ;
#34359=EDGE_CURVE ( 'NONE', #7716, #2811, #7130, .T. ) ;
#34451=CIRCLE ( 'NONE', #22524, 5.738084889453667792 ) ;
#34455=CARTESIAN_POINT ( 'NONE',  ( 212.5000000000000000, 0.000000000000000000, 7.500000000000000000 ) ) ;
#34473=CARTESIAN_POINT ( 'NONE',  ( 100.4534127715137544, -3.505526250977490488, 11.99932421786962244 ) ) ;
#34503=ORIENTED_EDGE ( 'NONE', *, *, #4110, .T. ) ;
#34558=CARTESIAN_POINT ( 'NONE',  ( 110.7380848894536598, -4.118294838564020743E-16, 7.500000000000000000 ) ) ;
#34576=DIRECTION ( 'NONE',  ( -1.000000000000000000, 0.000000000000000000, 0.000000000000000000 ) ) ;
#34606=EDGE_CURVE ( 'NONE', #5515, #31150, #33811, .T. ) ;
#34654=DIRECTION ( 'NONE',  ( -1.000000000000000000, 0.000000000000000000, 0.000000000000000000 ) ) ;
#34657=CARTESIAN_POINT ( 'NONE',  ( -105.3523586389574831, -5.105803102660850357, -5.493756281618515480 ) ) ;
#34684=DIRECTION ( 'NONE',  ( 1.000000000000000000, 0.000000000000000000, 0.000000000000000000 ) ) ;
#34694=CARTESIAN_POINT ( 'NONE',  ( 101.2263342230664591, -4.337494364694277849, 6.125882734748267389 ) ) ;
#34763=CARTESIAN_POINT ( 'NONE',  ( 105.7844661172050991, 5.687621871124707518, -4.888959764314519063 ) ) ;
#34765=CARTESIAN_POINT ( 'NONE',  ( -106.6936943766627053, 4.837773223901915998, -5.733537676439134145 ) ) ;
#34838=CARTESIAN_POINT ( 'NONE',  ( -102.4139082377428451, -4.424982940199789105, -6.059505149883824160 ) ) ;
#34923=CARTESIAN_POINT ( 'NONE',  ( 109.9370925636957139, 2.947297676519624599, 6.904853577595275738 ) ) ;
#34953=CARTESIAN_POINT ( 'NONE',  ( 103.6817977190026454, 5.587831648195836998, -11.18158713856774611 ) ) ;
#34962=ORIENTED_EDGE ( 'NONE', *, *, #26801, .F. ) ;
#34990=CARTESIAN_POINT ( 'NONE',  ( 212.5000000000000000, 0.000000000000000000, 0.000000000000000000 ) ) ;
#35016=CARTESIAN_POINT ( 'NONE',  ( -109.5736443501088928, -2.314419832420933520, -7.141071956987316227 ) ) ;
#35040=CARTESIAN_POINT ( 'NONE',  ( -104.6652972762545062, 5.115232524641492695, -11.40545467192879592 ) ) ;
#35084=EDGE_CURVE ( 'NONE', #10220, #14310, #31741, .T. ) ;
#35269=COLOUR_RGB('Grey',0.48,0.52,0.57);
#35270=FILL_AREA_STYLE_COLOUR('',#35269);
#35271=FILL_AREA_STYLE('',(#35270));
#35272=SURFACE_STYLE_FILL_AREA(#35271);
#35273=SURFACE_SIDE_STYLE('',(#35272));
#35274=SURFACE_STYLE_USAGE(.BOTH.,#35273);
#35275=PRESENTATION_STYLE_ASSIGNMENT((#35274));
ENDSEC;
END-ISO-10303-21;
